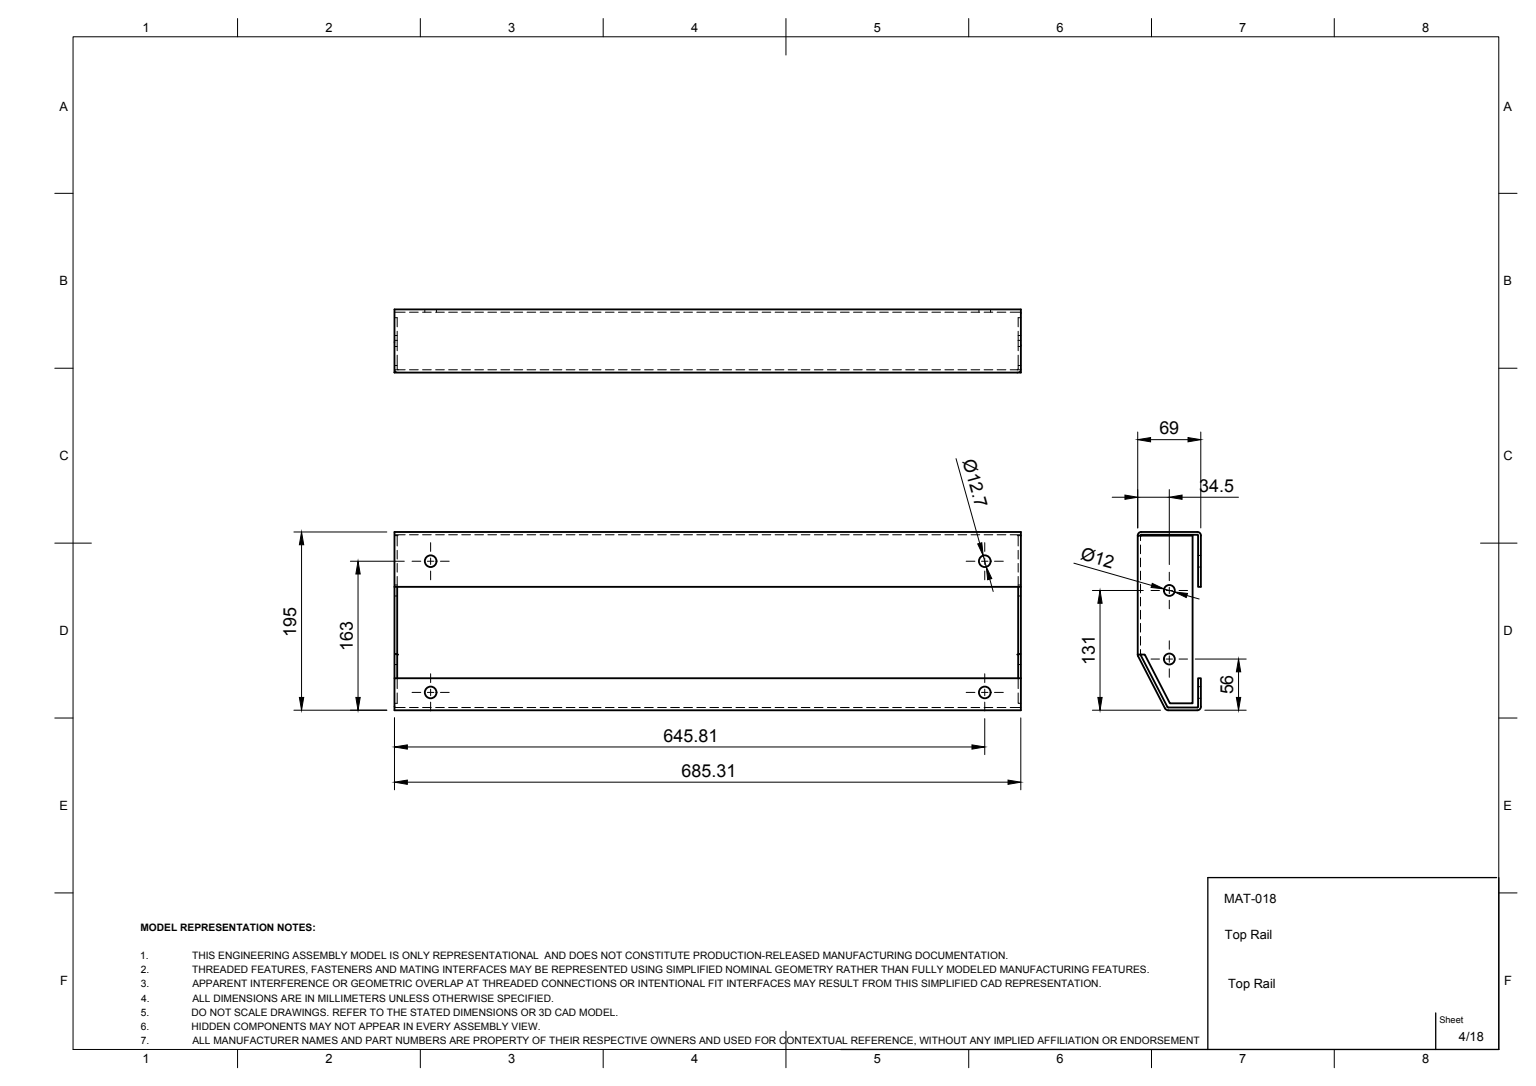
ISO-10303-21;
HEADER;
/* Generated by software containing ST-Developer
 * from STEP Tools, Inc. (www.steptools.com) 
 */

FILE_DESCRIPTION(
/* description */ ('STEP AP214'),
/* implementation_level */ '2;1');

FILE_NAME(
/* name */ 'Top Rail.step',
/* time_stamp */ '2026-11-14T06:16:09-08:00',
/* author */ (''),
/* organization */ (''),
/* preprocessor_version */ 'ST-DEVELOPER v20.2',
/* originating_system */ 'Autodesk Translation Framework v15.17.0.0',
/* authorisation */ '');

FILE_SCHEMA (('AUTOMOTIVE_DESIGN { 1 0 10303 214 3 1 1 }'));
ENDSEC;

DATA;
#10=MECHANICAL_DESIGN_GEOMETRIC_PRESENTATION_REPRESENTATION('',(#348),#18006);
#316=SHAPE_REPRESENTATION_RELATIONSHIP('SRR','None',#18072,#332);
#332=ADVANCED_BREP_SHAPE_REPRESENTATION('',(#364),#17989);
#348=STYLED_ITEM('',(#18170),#364);
#364=MANIFOLD_SOLID_BREP('Body1',#9557);
#401=FACE_BOUND('',#1553,.T.);
#402=FACE_BOUND('',#1554,.T.);
#403=FACE_BOUND('',#1557,.T.);
#404=FACE_BOUND('',#1558,.T.);
#405=FACE_BOUND('',#1568,.T.);
#406=FACE_BOUND('',#1569,.T.);
#407=FACE_BOUND('',#1572,.T.);
#408=FACE_BOUND('',#1573,.T.);
#409=FACE_BOUND('',#1591,.T.);
#410=FACE_BOUND('',#1592,.T.);
#411=FACE_BOUND('',#1594,.T.);
#412=FACE_BOUND('',#1595,.T.);
#413=FACE_BOUND('',#1606,.T.);
#414=FACE_BOUND('',#1607,.T.);
#415=FACE_BOUND('',#1609,.T.);
#416=FACE_BOUND('',#1610,.T.);
#558=PLANE('',#9911);
#559=PLANE('',#9913);
#560=PLANE('',#9915);
#561=PLANE('',#9916);
#562=PLANE('',#9917);
#563=PLANE('',#9919);
#564=PLANE('',#9921);
#565=PLANE('',#9924);
#566=PLANE('',#9925);
#567=PLANE('',#9928);
#568=PLANE('',#9929);
#569=PLANE('',#9932);
#570=PLANE('',#9935);
#571=PLANE('',#9936);
#572=PLANE('',#9939);
#573=PLANE('',#9940);
#574=PLANE('',#9943);
#575=PLANE('',#9946);
#576=PLANE('',#9947);
#577=PLANE('',#9950);
#578=PLANE('',#9951);
#579=PLANE('',#9954);
#580=PLANE('',#9955);
#581=PLANE('',#9958);
#582=PLANE('',#9959);
#583=PLANE('',#9960);
#584=PLANE('',#9961);
#585=PLANE('',#9963);
#586=PLANE('',#9965);
#587=PLANE('',#9968);
#588=PLANE('',#9970);
#589=PLANE('',#9971);
#590=PLANE('',#9972);
#591=PLANE('',#9974);
#592=PLANE('',#9977);
#593=PLANE('',#9979);
#594=PLANE('',#9981);
#595=PLANE('',#9982);
#596=PLANE('',#9983);
#597=PLANE('',#9986);
#598=PLANE('',#9991);
#599=PLANE('',#9992);
#600=PLANE('',#9993);
#601=PLANE('',#9994);
#602=PLANE('',#9995);
#603=PLANE('',#9996);
#604=PLANE('',#9997);
#605=PLANE('',#9998);
#606=PLANE('',#10001);
#607=PLANE('',#10006);
#608=PLANE('',#10007);
#609=PLANE('',#10008);
#610=PLANE('',#10009);
#611=PLANE('',#10010);
#612=PLANE('',#10011);
#613=PLANE('',#10012);
#922=FACE_OUTER_BOUND('',#1520,.T.);
#923=FACE_OUTER_BOUND('',#1521,.T.);
#924=FACE_OUTER_BOUND('',#1522,.T.);
#925=FACE_OUTER_BOUND('',#1523,.T.);
#926=FACE_OUTER_BOUND('',#1524,.T.);
#927=FACE_OUTER_BOUND('',#1525,.T.);
#928=FACE_OUTER_BOUND('',#1526,.T.);
#929=FACE_OUTER_BOUND('',#1527,.T.);
#930=FACE_OUTER_BOUND('',#1528,.T.);
#931=FACE_OUTER_BOUND('',#1529,.T.);
#932=FACE_OUTER_BOUND('',#1530,.T.);
#933=FACE_OUTER_BOUND('',#1531,.T.);
#934=FACE_OUTER_BOUND('',#1532,.T.);
#935=FACE_OUTER_BOUND('',#1533,.T.);
#936=FACE_OUTER_BOUND('',#1534,.T.);
#937=FACE_OUTER_BOUND('',#1535,.T.);
#938=FACE_OUTER_BOUND('',#1536,.T.);
#939=FACE_OUTER_BOUND('',#1537,.T.);
#940=FACE_OUTER_BOUND('',#1538,.T.);
#941=FACE_OUTER_BOUND('',#1539,.T.);
#942=FACE_OUTER_BOUND('',#1540,.T.);
#943=FACE_OUTER_BOUND('',#1541,.T.);
#944=FACE_OUTER_BOUND('',#1542,.T.);
#945=FACE_OUTER_BOUND('',#1543,.T.);
#946=FACE_OUTER_BOUND('',#1544,.T.);
#947=FACE_OUTER_BOUND('',#1545,.T.);
#948=FACE_OUTER_BOUND('',#1546,.T.);
#949=FACE_OUTER_BOUND('',#1547,.T.);
#950=FACE_OUTER_BOUND('',#1548,.T.);
#951=FACE_OUTER_BOUND('',#1549,.T.);
#952=FACE_OUTER_BOUND('',#1550,.T.);
#953=FACE_OUTER_BOUND('',#1551,.T.);
#954=FACE_OUTER_BOUND('',#1552,.T.);
#955=FACE_OUTER_BOUND('',#1555,.T.);
#956=FACE_OUTER_BOUND('',#1556,.T.);
#957=FACE_OUTER_BOUND('',#1559,.T.);
#958=FACE_OUTER_BOUND('',#1560,.T.);
#959=FACE_OUTER_BOUND('',#1561,.T.);
#960=FACE_OUTER_BOUND('',#1562,.T.);
#961=FACE_OUTER_BOUND('',#1563,.T.);
#962=FACE_OUTER_BOUND('',#1564,.T.);
#963=FACE_OUTER_BOUND('',#1565,.T.);
#964=FACE_OUTER_BOUND('',#1566,.T.);
#965=FACE_OUTER_BOUND('',#1567,.T.);
#966=FACE_OUTER_BOUND('',#1570,.T.);
#967=FACE_OUTER_BOUND('',#1571,.T.);
#968=FACE_OUTER_BOUND('',#1574,.T.);
#969=FACE_OUTER_BOUND('',#1575,.T.);
#970=FACE_OUTER_BOUND('',#1576,.T.);
#971=FACE_OUTER_BOUND('',#1577,.T.);
#972=FACE_OUTER_BOUND('',#1578,.T.);
#973=FACE_OUTER_BOUND('',#1579,.T.);
#974=FACE_OUTER_BOUND('',#1580,.T.);
#975=FACE_OUTER_BOUND('',#1581,.T.);
#976=FACE_OUTER_BOUND('',#1582,.T.);
#977=FACE_OUTER_BOUND('',#1583,.T.);
#978=FACE_OUTER_BOUND('',#1584,.T.);
#979=FACE_OUTER_BOUND('',#1585,.T.);
#980=FACE_OUTER_BOUND('',#1586,.T.);
#981=FACE_OUTER_BOUND('',#1587,.T.);
#982=FACE_OUTER_BOUND('',#1588,.T.);
#983=FACE_OUTER_BOUND('',#1589,.T.);
#984=FACE_OUTER_BOUND('',#1590,.T.);
#985=FACE_OUTER_BOUND('',#1593,.T.);
#986=FACE_OUTER_BOUND('',#1596,.T.);
#987=FACE_OUTER_BOUND('',#1597,.T.);
#988=FACE_OUTER_BOUND('',#1598,.T.);
#989=FACE_OUTER_BOUND('',#1599,.T.);
#990=FACE_OUTER_BOUND('',#1600,.T.);
#991=FACE_OUTER_BOUND('',#1601,.T.);
#992=FACE_OUTER_BOUND('',#1602,.T.);
#993=FACE_OUTER_BOUND('',#1603,.T.);
#994=FACE_OUTER_BOUND('',#1604,.T.);
#995=FACE_OUTER_BOUND('',#1605,.T.);
#996=FACE_OUTER_BOUND('',#1608,.T.);
#997=FACE_OUTER_BOUND('',#1611,.T.);
#998=FACE_OUTER_BOUND('',#1612,.T.);
#999=FACE_OUTER_BOUND('',#1613,.T.);
#1520=EDGE_LOOP('',(#6522,#6523,#6524,#6525));
#1521=EDGE_LOOP('',(#6526,#6527,#6528,#6529));
#1522=EDGE_LOOP('',(#6530,#6531,#6532,#6533));
#1523=EDGE_LOOP('',(#6534,#6535,#6536,#6537));
#1524=EDGE_LOOP('',(#6538,#6539,#6540,#6541));
#1525=EDGE_LOOP('',(#6542,#6543,#6544,#6545));
#1526=EDGE_LOOP('',(#6546,#6547,#6548,#6549));
#1527=EDGE_LOOP('',(#6550,#6551,#6552,#6553));
#1528=EDGE_LOOP('',(#6554,#6555,#6556,#6557));
#1529=EDGE_LOOP('',(#6558,#6559,#6560,#6561));
#1530=EDGE_LOOP('',(#6562,#6563,#6564,#6565));
#1531=EDGE_LOOP('',(#6566,#6567,#6568,#6569));
#1532=EDGE_LOOP('',(#6570,#6571,#6572,#6573));
#1533=EDGE_LOOP('',(#6574,#6575,#6576,#6577));
#1534=EDGE_LOOP('',(#6578,#6579,#6580,#6581));
#1535=EDGE_LOOP('',(#6582,#6583,#6584,#6585));
#1536=EDGE_LOOP('',(#6586,#6587,#6588,#6589));
#1537=EDGE_LOOP('',(#6590,#6591,#6592,#6593));
#1538=EDGE_LOOP('',(#6594,#6595,#6596,#6597));
#1539=EDGE_LOOP('',(#6598,#6599,#6600,#6601));
#1540=EDGE_LOOP('',(#6602,#6603,#6604,#6605));
#1541=EDGE_LOOP('',(#6606,#6607,#6608,#6609));
#1542=EDGE_LOOP('',(#6610,#6611,#6612,#6613));
#1543=EDGE_LOOP('',(#6614,#6615,#6616,#6617));
#1544=EDGE_LOOP('',(#6618,#6619,#6620,#6621));
#1545=EDGE_LOOP('',(#6622,#6623,#6624,#6625));
#1546=EDGE_LOOP('',(#6626,#6627,#6628,#6629));
#1547=EDGE_LOOP('',(#6630,#6631,#6632,#6633));
#1548=EDGE_LOOP('',(#6634,#6635,#6636,#6637));
#1549=EDGE_LOOP('',(#6638,#6639,#6640,#6641));
#1550=EDGE_LOOP('',(#6642,#6643,#6644,#6645));
#1551=EDGE_LOOP('',(#6646,#6647,#6648,#6649));
#1552=EDGE_LOOP('',(#6650,#6651,#6652,#6653));
#1553=EDGE_LOOP('',(#6654));
#1554=EDGE_LOOP('',(#6655));
#1555=EDGE_LOOP('',(#6656,#6657,#6658,#6659));
#1556=EDGE_LOOP('',(#6660,#6661,#6662,#6663));
#1557=EDGE_LOOP('',(#6664));
#1558=EDGE_LOOP('',(#6665));
#1559=EDGE_LOOP('',(#6666,#6667,#6668,#6669));
#1560=EDGE_LOOP('',(#6670,#6671,#6672,#6673));
#1561=EDGE_LOOP('',(#6674,#6675,#6676,#6677));
#1562=EDGE_LOOP('',(#6678,#6679,#6680,#6681));
#1563=EDGE_LOOP('',(#6682,#6683,#6684,#6685,#6686,#6687));
#1564=EDGE_LOOP('',(#6688,#6689,#6690,#6691,#6692,#6693));
#1565=EDGE_LOOP('',(#6694,#6695,#6696,#6697));
#1566=EDGE_LOOP('',(#6698,#6699,#6700,#6701));
#1567=EDGE_LOOP('',(#6702,#6703,#6704,#6705));
#1568=EDGE_LOOP('',(#6706));
#1569=EDGE_LOOP('',(#6707));
#1570=EDGE_LOOP('',(#6708,#6709,#6710,#6711));
#1571=EDGE_LOOP('',(#6712,#6713,#6714,#6715));
#1572=EDGE_LOOP('',(#6716));
#1573=EDGE_LOOP('',(#6717));
#1574=EDGE_LOOP('',(#6718,#6719,#6720,#6721));
#1575=EDGE_LOOP('',(#6722,#6723,#6724,#6725));
#1576=EDGE_LOOP('',(#6726,#6727,#6728,#6729,#6730,#6731,#6732,#6733));
#1577=EDGE_LOOP('',(#6734,#6735,#6736,#6737,#6738,#6739,#6740,#6741));
#1578=EDGE_LOOP('',(#6742,#6743,#6744,#6745));
#1579=EDGE_LOOP('',(#6746,#6747,#6748,#6749));
#1580=EDGE_LOOP('',(#6750,#6751,#6752,#6753));
#1581=EDGE_LOOP('',(#6754,#6755,#6756,#6757));
#1582=EDGE_LOOP('',(#6758,#6759,#6760,#6761));
#1583=EDGE_LOOP('',(#6762,#6763,#6764,#6765));
#1584=EDGE_LOOP('',(#6766,#6767,#6768,#6769));
#1585=EDGE_LOOP('',(#6770,#6771,#6772,#6773));
#1586=EDGE_LOOP('',(#6774,#6775,#6776,#6777,#6778,#6779));
#1587=EDGE_LOOP('',(#6780,#6781,#6782,#6783));
#1588=EDGE_LOOP('',(#6784,#6785,#6786,#6787));
#1589=EDGE_LOOP('',(#6788,#6789,#6790,#6791));
#1590=EDGE_LOOP('',(#6792,#6793,#6794,#6795,#6796,#6797));
#1591=EDGE_LOOP('',(#6798));
#1592=EDGE_LOOP('',(#6799));
#1593=EDGE_LOOP('',(#6800,#6801,#6802,#6803,#6804,#6805));
#1594=EDGE_LOOP('',(#6806));
#1595=EDGE_LOOP('',(#6807));
#1596=EDGE_LOOP('',(#6808,#6809,#6810,#6811));
#1597=EDGE_LOOP('',(#6812,#6813,#6814,#6815));
#1598=EDGE_LOOP('',(#6816,#6817,#6818,#6819));
#1599=EDGE_LOOP('',(#6820,#6821,#6822,#6823));
#1600=EDGE_LOOP('',(#6824,#6825,#6826,#6827));
#1601=EDGE_LOOP('',(#6828,#6829,#6830,#6831,#6832,#6833));
#1602=EDGE_LOOP('',(#6834,#6835,#6836,#6837));
#1603=EDGE_LOOP('',(#6838,#6839,#6840,#6841));
#1604=EDGE_LOOP('',(#6842,#6843,#6844,#6845));
#1605=EDGE_LOOP('',(#6846,#6847,#6848,#6849,#6850,#6851));
#1606=EDGE_LOOP('',(#6852));
#1607=EDGE_LOOP('',(#6853));
#1608=EDGE_LOOP('',(#6854,#6855,#6856,#6857,#6858,#6859));
#1609=EDGE_LOOP('',(#6860));
#1610=EDGE_LOOP('',(#6861));
#1611=EDGE_LOOP('',(#6862,#6863,#6864,#6865));
#1612=EDGE_LOOP('',(#6866,#6867,#6868,#6869));
#1613=EDGE_LOOP('',(#6870,#6871,#6872,#6873));
#2247=LINE('',#14188,#2971);
#2248=LINE('',#14194,#2972);
#2249=LINE('',#14200,#2973);
#2250=LINE('',#14206,#2974);
#2251=LINE('',#14212,#2975);
#2252=LINE('',#14218,#2976);
#2253=LINE('',#14224,#2977);
#2254=LINE('',#14230,#2978);
#2255=LINE('',#14235,#2979);
#2256=LINE('',#14239,#2980);
#2257=LINE('',#14240,#2981);
#2258=LINE('',#14244,#2982);
#2259=LINE('',#14248,#2983);
#2260=LINE('',#14249,#2984);
#2261=LINE('',#14252,#2985);
#2262=LINE('',#14253,#2986);
#2263=LINE('',#14255,#2987);
#2264=LINE('',#14256,#2988);
#2265=LINE('',#14260,#2989);
#2266=LINE('',#14262,#2990);
#2267=LINE('',#14264,#2991);
#2268=LINE('',#14265,#2992);
#2269=LINE('',#14269,#2993);
#2270=LINE('',#14272,#2994);
#2271=LINE('',#14273,#2995);
#2272=LINE('',#14276,#2996);
#2273=LINE('',#14280,#2997);
#2274=LINE('',#14281,#2998);
#2275=LINE('',#14285,#2999);
#2276=LINE('',#14289,#3000);
#2277=LINE('',#14293,#3001);
#2278=LINE('',#14295,#3002);
#2279=LINE('',#14296,#3003);
#2280=LINE('',#14300,#3004);
#2281=LINE('',#14304,#3005);
#2282=LINE('',#14308,#3006);
#2283=LINE('',#14310,#3007);
#2284=LINE('',#14311,#3008);
#2285=LINE('',#14318,#3009);
#2286=LINE('',#14322,#3010);
#2287=LINE('',#14323,#3011);
#2288=LINE('',#14327,#3012);
#2289=LINE('',#14332,#3013);
#2290=LINE('',#14334,#3014);
#2291=LINE('',#14335,#3015);
#2292=LINE('',#14340,#3016);
#2293=LINE('',#14345,#3017);
#2294=LINE('',#14350,#3018);
#2295=LINE('',#14352,#3019);
#2296=LINE('',#14353,#3020);
#2297=LINE('',#14357,#3021);
#2298=LINE('',#14361,#3022);
#2299=LINE('',#14364,#3023);
#2300=LINE('',#14365,#3024);
#2301=LINE('',#14369,#3025);
#2302=LINE('',#14374,#3026);
#2303=LINE('',#14376,#3027);
#2304=LINE('',#14377,#3028);
#2305=LINE('',#14381,#3029);
#2306=LINE('',#14385,#3030);
#2307=LINE('',#14388,#3031);
#2308=LINE('',#14389,#3032);
#2309=LINE('',#14392,#3033);
#2310=LINE('',#14393,#3034);
#2311=LINE('',#14394,#3035);
#2312=LINE('',#14397,#3036);
#2313=LINE('',#14398,#3037);
#2314=LINE('',#14400,#3038);
#2315=LINE('',#14401,#3039);
#2316=LINE('',#14403,#3040);
#2317=LINE('',#14405,#3041);
#2318=LINE('',#14407,#3042);
#2319=LINE('',#14409,#3043);
#2320=LINE('',#14412,#3044);
#2321=LINE('',#14414,#3045);
#2322=LINE('',#14416,#3046);
#2323=LINE('',#14419,#3047);
#2324=LINE('',#14420,#3048);
#2325=LINE('',#14423,#3049);
#2326=LINE('',#14424,#3050);
#2327=LINE('',#14426,#3051);
#2328=LINE('',#14427,#3052);
#2329=LINE('',#14429,#3053);
#2330=LINE('',#14431,#3054);
#2331=LINE('',#14433,#3055);
#2332=LINE('',#14434,#3056);
#2333=LINE('',#14436,#3057);
#2334=LINE('',#14437,#3058);
#2335=LINE('',#14438,#3059);
#2336=LINE('',#14440,#3060);
#2337=LINE('',#14442,#3061);
#2338=LINE('',#14444,#3062);
#2339=LINE('',#14452,#3063);
#2340=LINE('',#14459,#3064);
#2341=LINE('',#14461,#3065);
#2342=LINE('',#14463,#3066);
#2343=LINE('',#14466,#3067);
#2344=LINE('',#14468,#3068);
#2345=LINE('',#14469,#3069);
#2346=LINE('',#14472,#3070);
#2347=LINE('',#14474,#3071);
#2348=LINE('',#14475,#3072);
#2349=LINE('',#14478,#3073);
#2350=LINE('',#14480,#3074);
#2351=LINE('',#14481,#3075);
#2352=LINE('',#14484,#3076);
#2353=LINE('',#14486,#3077);
#2354=LINE('',#14487,#3078);
#2355=LINE('',#14489,#3079);
#2356=LINE('',#14491,#3080);
#2357=LINE('',#14498,#3081);
#2358=LINE('',#14504,#3082);
#2359=LINE('',#14506,#3083);
#2360=LINE('',#14508,#3084);
#2361=LINE('',#14511,#3085);
#2362=LINE('',#14513,#3086);
#2363=LINE('',#14514,#3087);
#2364=LINE('',#14517,#3088);
#2365=LINE('',#14519,#3089);
#2366=LINE('',#14520,#3090);
#2367=LINE('',#14523,#3091);
#2368=LINE('',#14525,#3092);
#2369=LINE('',#14526,#3093);
#2370=LINE('',#14529,#3094);
#2371=LINE('',#14531,#3095);
#2372=LINE('',#14532,#3096);
#2373=LINE('',#14534,#3097);
#2374=LINE('',#14536,#3098);
#2971=VECTOR('',#11272,6.00000000000001);
#2972=VECTOR('',#11279,6.00000000000001);
#2973=VECTOR('',#11286,6.00000000000001);
#2974=VECTOR('',#11293,6.00000000000001);
#2975=VECTOR('',#11300,6.34999999999994);
#2976=VECTOR('',#11307,6.34999999999997);
#2977=VECTOR('',#11314,6.34999999999995);
#2978=VECTOR('',#11321,6.34999999999997);
#2979=VECTOR('',#11326,1000.);
#2980=VECTOR('',#11329,1000.);
#2981=VECTOR('',#11330,1000.);
#2982=VECTOR('',#11333,1000.);
#2983=VECTOR('',#11336,1000.);
#2984=VECTOR('',#11337,1000.);
#2985=VECTOR('',#11340,1000.);
#2986=VECTOR('',#11341,1000.);
#2987=VECTOR('',#11342,1000.);
#2988=VECTOR('',#11343,1000.);
#2989=VECTOR('',#11346,1000.);
#2990=VECTOR('',#11347,1000.);
#2991=VECTOR('',#11348,1000.);
#2992=VECTOR('',#11349,1000.);
#2993=VECTOR('',#11352,1000.);
#2994=VECTOR('',#11355,1000.);
#2995=VECTOR('',#11356,1000.);
#2996=VECTOR('',#11359,1000.);
#2997=VECTOR('',#11362,1000.);
#2998=VECTOR('',#11363,1000.);
#2999=VECTOR('',#11366,1000.);
#3000=VECTOR('',#11369,1000.);
#3001=VECTOR('',#11374,1000.);
#3002=VECTOR('',#11375,1000.);
#3003=VECTOR('',#11376,1000.);
#3004=VECTOR('',#11379,1000.);
#3005=VECTOR('',#11382,1000.);
#3006=VECTOR('',#11387,1000.);
#3007=VECTOR('',#11388,1000.);
#3008=VECTOR('',#11389,1000.);
#3009=VECTOR('',#11398,1000.);
#3010=VECTOR('',#11405,1000.);
#3011=VECTOR('',#11406,1000.);
#3012=VECTOR('',#11409,1000.);
#3013=VECTOR('',#11416,1000.);
#3014=VECTOR('',#11417,1000.);
#3015=VECTOR('',#11418,1000.);
#3016=VECTOR('',#11423,1000.);
#3017=VECTOR('',#11428,1000.);
#3018=VECTOR('',#11435,1000.);
#3019=VECTOR('',#11436,1000.);
#3020=VECTOR('',#11437,1000.);
#3021=VECTOR('',#11440,1000.);
#3022=VECTOR('',#11443,1000.);
#3023=VECTOR('',#11448,1000.);
#3024=VECTOR('',#11449,1000.);
#3025=VECTOR('',#11452,1000.);
#3026=VECTOR('',#11459,1000.);
#3027=VECTOR('',#11460,1000.);
#3028=VECTOR('',#11461,1000.);
#3029=VECTOR('',#11464,1000.);
#3030=VECTOR('',#11467,1000.);
#3031=VECTOR('',#11472,1000.);
#3032=VECTOR('',#11473,1000.);
#3033=VECTOR('',#11476,1000.);
#3034=VECTOR('',#11477,1000.);
#3035=VECTOR('',#11478,1000.);
#3036=VECTOR('',#11481,1000.);
#3037=VECTOR('',#11482,1000.);
#3038=VECTOR('',#11485,1000.);
#3039=VECTOR('',#11486,1000.);
#3040=VECTOR('',#11489,1000.);
#3041=VECTOR('',#11492,1000.);
#3042=VECTOR('',#11495,1000.);
#3043=VECTOR('',#11498,1000.);
#3044=VECTOR('',#11503,1000.);
#3045=VECTOR('',#11506,1000.);
#3046=VECTOR('',#11509,1000.);
#3047=VECTOR('',#11512,1000.);
#3048=VECTOR('',#11513,1000.);
#3049=VECTOR('',#11516,1000.);
#3050=VECTOR('',#11517,1000.);
#3051=VECTOR('',#11520,1000.);
#3052=VECTOR('',#11521,1000.);
#3053=VECTOR('',#11524,1000.);
#3054=VECTOR('',#11527,1000.);
#3055=VECTOR('',#11530,1000.);
#3056=VECTOR('',#11531,1000.);
#3057=VECTOR('',#11534,1000.);
#3058=VECTOR('',#11535,1000.);
#3059=VECTOR('',#11536,1000.);
#3060=VECTOR('',#11539,1000.);
#3061=VECTOR('',#11542,1000.);
#3062=VECTOR('',#11545,1000.);
#3063=VECTOR('',#11556,1000.);
#3064=VECTOR('',#11565,1000.);
#3065=VECTOR('',#11568,1000.);
#3066=VECTOR('',#11571,1000.);
#3067=VECTOR('',#11574,1000.);
#3068=VECTOR('',#11575,1000.);
#3069=VECTOR('',#11576,1000.);
#3070=VECTOR('',#11579,1000.);
#3071=VECTOR('',#11580,1000.);
#3072=VECTOR('',#11581,1000.);
#3073=VECTOR('',#11584,1000.);
#3074=VECTOR('',#11585,1000.);
#3075=VECTOR('',#11586,1000.);
#3076=VECTOR('',#11589,1000.);
#3077=VECTOR('',#11590,1000.);
#3078=VECTOR('',#11591,1000.);
#3079=VECTOR('',#11594,1000.);
#3080=VECTOR('',#11597,1000.);
#3081=VECTOR('',#11606,1000.);
#3082=VECTOR('',#11613,1000.);
#3083=VECTOR('',#11616,1000.);
#3084=VECTOR('',#11619,1000.);
#3085=VECTOR('',#11622,1000.);
#3086=VECTOR('',#11623,1000.);
#3087=VECTOR('',#11624,1000.);
#3088=VECTOR('',#11627,1000.);
#3089=VECTOR('',#11628,1000.);
#3090=VECTOR('',#11629,1000.);
#3091=VECTOR('',#11632,1000.);
#3092=VECTOR('',#11633,1000.);
#3093=VECTOR('',#11634,1000.);
#3094=VECTOR('',#11637,1000.);
#3095=VECTOR('',#11638,1000.);
#3096=VECTOR('',#11639,1000.);
#3097=VECTOR('',#11642,1000.);
#3098=VECTOR('',#11645,1000.);
#3618=CIRCLE('',#9888,6.00000000000001);
#3619=CIRCLE('',#9889,6.00000000000001);
#3620=CIRCLE('',#9891,6.00000000000002);
#3621=CIRCLE('',#9892,6.00000000000001);
#3622=CIRCLE('',#9894,6.00000000000001);
#3623=CIRCLE('',#9895,6.00000000000001);
#3624=CIRCLE('',#9897,6.00000000000001);
#3625=CIRCLE('',#9898,6.00000000000002);
#3626=CIRCLE('',#9900,6.34999999999994);
#3627=CIRCLE('',#9901,6.34999999999994);
#3628=CIRCLE('',#9903,6.34999999999994);
#3629=CIRCLE('',#9904,6.34999999999997);
#3630=CIRCLE('',#9906,6.34999999999995);
#3631=CIRCLE('',#9907,6.34999999999995);
#3632=CIRCLE('',#9909,6.34999999999997);
#3633=CIRCLE('',#9910,6.34999999999997);
#3634=CIRCLE('',#9912,4.);
#3635=CIRCLE('',#9914,4.);
#3636=CIRCLE('',#9918,4.);
#3637=CIRCLE('',#9920,4.);
#3638=CIRCLE('',#9922,4.);
#3639=CIRCLE('',#9923,1.);
#3640=CIRCLE('',#9926,4.);
#3641=CIRCLE('',#9927,1.);
#3642=CIRCLE('',#9930,4.);
#3643=CIRCLE('',#9931,1.);
#3644=CIRCLE('',#9933,4.);
#3645=CIRCLE('',#9934,1.);
#3646=CIRCLE('',#9937,4.);
#3647=CIRCLE('',#9938,1.);
#3648=CIRCLE('',#9941,4.);
#3649=CIRCLE('',#9942,1.);
#3650=CIRCLE('',#9944,4.);
#3651=CIRCLE('',#9945,1.);
#3652=CIRCLE('',#9948,4.);
#3653=CIRCLE('',#9949,1.);
#3654=CIRCLE('',#9952,4.);
#3655=CIRCLE('',#9953,1.);
#3656=CIRCLE('',#9956,4.);
#3657=CIRCLE('',#9957,1.);
#3658=CIRCLE('',#9984,4.);
#3659=CIRCLE('',#9985,1.);
#3660=CIRCLE('',#9987,4.);
#3661=CIRCLE('',#9988,1.);
#3662=CIRCLE('',#9999,1.);
#3663=CIRCLE('',#10000,4.);
#3664=CIRCLE('',#10002,4.);
#3665=CIRCLE('',#10003,1.);
#4119=VERTEX_POINT('',#14185);
#4120=VERTEX_POINT('',#14187);
#4121=VERTEX_POINT('',#14191);
#4122=VERTEX_POINT('',#14193);
#4123=VERTEX_POINT('',#14197);
#4124=VERTEX_POINT('',#14199);
#4125=VERTEX_POINT('',#14203);
#4126=VERTEX_POINT('',#14205);
#4127=VERTEX_POINT('',#14209);
#4128=VERTEX_POINT('',#14211);
#4129=VERTEX_POINT('',#14215);
#4130=VERTEX_POINT('',#14217);
#4131=VERTEX_POINT('',#14221);
#4132=VERTEX_POINT('',#14223);
#4133=VERTEX_POINT('',#14227);
#4134=VERTEX_POINT('',#14229);
#4135=VERTEX_POINT('',#14233);
#4136=VERTEX_POINT('',#14234);
#4137=VERTEX_POINT('',#14236);
#4138=VERTEX_POINT('',#14238);
#4139=VERTEX_POINT('',#14242);
#4140=VERTEX_POINT('',#14243);
#4141=VERTEX_POINT('',#14245);
#4142=VERTEX_POINT('',#14247);
#4143=VERTEX_POINT('',#14251);
#4144=VERTEX_POINT('',#14254);
#4145=VERTEX_POINT('',#14258);
#4146=VERTEX_POINT('',#14259);
#4147=VERTEX_POINT('',#14261);
#4148=VERTEX_POINT('',#14263);
#4149=VERTEX_POINT('',#14267);
#4150=VERTEX_POINT('',#14268);
#4151=VERTEX_POINT('',#14271);
#4152=VERTEX_POINT('',#14275);
#4153=VERTEX_POINT('',#14277);
#4154=VERTEX_POINT('',#14279);
#4155=VERTEX_POINT('',#14283);
#4156=VERTEX_POINT('',#14284);
#4157=VERTEX_POINT('',#14286);
#4158=VERTEX_POINT('',#14288);
#4159=VERTEX_POINT('',#14292);
#4160=VERTEX_POINT('',#14294);
#4161=VERTEX_POINT('',#14298);
#4162=VERTEX_POINT('',#14299);
#4163=VERTEX_POINT('',#14301);
#4164=VERTEX_POINT('',#14303);
#4165=VERTEX_POINT('',#14307);
#4166=VERTEX_POINT('',#14309);
#4167=VERTEX_POINT('',#14316);
#4168=VERTEX_POINT('',#14317);
#4169=VERTEX_POINT('',#14325);
#4170=VERTEX_POINT('',#14326);
#4171=VERTEX_POINT('',#14331);
#4172=VERTEX_POINT('',#14333);
#4173=VERTEX_POINT('',#14337);
#4174=VERTEX_POINT('',#14339);
#4175=VERTEX_POINT('',#14343);
#4176=VERTEX_POINT('',#14344);
#4177=VERTEX_POINT('',#14349);
#4178=VERTEX_POINT('',#14351);
#4179=VERTEX_POINT('',#14355);
#4180=VERTEX_POINT('',#14356);
#4181=VERTEX_POINT('',#14358);
#4182=VERTEX_POINT('',#14360);
#4183=VERTEX_POINT('',#14367);
#4184=VERTEX_POINT('',#14368);
#4185=VERTEX_POINT('',#14373);
#4186=VERTEX_POINT('',#14375);
#4187=VERTEX_POINT('',#14379);
#4188=VERTEX_POINT('',#14380);
#4189=VERTEX_POINT('',#14382);
#4190=VERTEX_POINT('',#14384);
#4191=VERTEX_POINT('',#14391);
#4192=VERTEX_POINT('',#14396);
#4193=VERTEX_POINT('',#14418);
#4194=VERTEX_POINT('',#14422);
#4195=VERTEX_POINT('',#14449);
#4196=VERTEX_POINT('',#14451);
#4197=VERTEX_POINT('',#14455);
#4198=VERTEX_POINT('',#14457);
#4199=VERTEX_POINT('',#14465);
#4200=VERTEX_POINT('',#14467);
#4201=VERTEX_POINT('',#14471);
#4202=VERTEX_POINT('',#14473);
#4203=VERTEX_POINT('',#14477);
#4204=VERTEX_POINT('',#14479);
#4205=VERTEX_POINT('',#14483);
#4206=VERTEX_POINT('',#14485);
#4207=VERTEX_POINT('',#14494);
#4208=VERTEX_POINT('',#14496);
#4209=VERTEX_POINT('',#14500);
#4210=VERTEX_POINT('',#14502);
#4211=VERTEX_POINT('',#14510);
#4212=VERTEX_POINT('',#14512);
#4213=VERTEX_POINT('',#14516);
#4214=VERTEX_POINT('',#14518);
#4215=VERTEX_POINT('',#14522);
#4216=VERTEX_POINT('',#14524);
#4217=VERTEX_POINT('',#14528);
#4218=VERTEX_POINT('',#14530);
#5009=EDGE_CURVE('',#4119,#4119,#3618,.T.);
#5010=EDGE_CURVE('',#4119,#4120,#2247,.T.);
#5011=EDGE_CURVE('',#4120,#4120,#3619,.T.);
#5012=EDGE_CURVE('',#4121,#4121,#3620,.T.);
#5013=EDGE_CURVE('',#4121,#4122,#2248,.T.);
#5014=EDGE_CURVE('',#4122,#4122,#3621,.T.);
#5015=EDGE_CURVE('',#4123,#4123,#3622,.T.);
#5016=EDGE_CURVE('',#4123,#4124,#2249,.T.);
#5017=EDGE_CURVE('',#4124,#4124,#3623,.T.);
#5018=EDGE_CURVE('',#4125,#4125,#3624,.T.);
#5019=EDGE_CURVE('',#4125,#4126,#2250,.T.);
#5020=EDGE_CURVE('',#4126,#4126,#3625,.T.);
#5021=EDGE_CURVE('',#4127,#4127,#3626,.T.);
#5022=EDGE_CURVE('',#4127,#4128,#2251,.T.);
#5023=EDGE_CURVE('',#4128,#4128,#3627,.T.);
#5024=EDGE_CURVE('',#4129,#4129,#3628,.T.);
#5025=EDGE_CURVE('',#4129,#4130,#2252,.T.);
#5026=EDGE_CURVE('',#4130,#4130,#3629,.T.);
#5027=EDGE_CURVE('',#4131,#4131,#3630,.T.);
#5028=EDGE_CURVE('',#4131,#4132,#2253,.T.);
#5029=EDGE_CURVE('',#4132,#4132,#3631,.T.);
#5030=EDGE_CURVE('',#4133,#4133,#3632,.T.);
#5031=EDGE_CURVE('',#4133,#4134,#2254,.T.);
#5032=EDGE_CURVE('',#4134,#4134,#3633,.T.);
#5033=EDGE_CURVE('',#4135,#4136,#2255,.T.);
#5034=EDGE_CURVE('',#4136,#4137,#3634,.T.);
#5035=EDGE_CURVE('',#4138,#4137,#2256,.T.);
#5036=EDGE_CURVE('',#4138,#4135,#2257,.T.);
#5037=EDGE_CURVE('',#4139,#4140,#2258,.T.);
#5038=EDGE_CURVE('',#4139,#4141,#3635,.T.);
#5039=EDGE_CURVE('',#4141,#4142,#2259,.T.);
#5040=EDGE_CURVE('',#4142,#4140,#2260,.T.);
#5041=EDGE_CURVE('',#4143,#4137,#2261,.T.);
#5042=EDGE_CURVE('',#4137,#4139,#2262,.T.);
#5043=EDGE_CURVE('',#4144,#4139,#2263,.T.);
#5044=EDGE_CURVE('',#4144,#4143,#2264,.T.);
#5045=EDGE_CURVE('',#4145,#4146,#2265,.T.);
#5046=EDGE_CURVE('',#4147,#4145,#2266,.T.);
#5047=EDGE_CURVE('',#4148,#4147,#2267,.T.);
#5048=EDGE_CURVE('',#4148,#4146,#2268,.T.);
#5049=EDGE_CURVE('',#4149,#4150,#2269,.T.);
#5050=EDGE_CURVE('',#4150,#4144,#3636,.T.);
#5051=EDGE_CURVE('',#4151,#4144,#2270,.T.);
#5052=EDGE_CURVE('',#4151,#4149,#2271,.T.);
#5053=EDGE_CURVE('',#4152,#4143,#2272,.T.);
#5054=EDGE_CURVE('',#4143,#4153,#3637,.T.);
#5055=EDGE_CURVE('',#4154,#4153,#2273,.T.);
#5056=EDGE_CURVE('',#4154,#4152,#2274,.T.);
#5057=EDGE_CURVE('',#4155,#4156,#2275,.T.);
#5058=EDGE_CURVE('',#4157,#4155,#3638,.T.);
#5059=EDGE_CURVE('',#4158,#4157,#2276,.T.);
#5060=EDGE_CURVE('',#4158,#4156,#3639,.T.);
#5061=EDGE_CURVE('',#4155,#4159,#2277,.T.);
#5062=EDGE_CURVE('',#4156,#4160,#2278,.T.);
#5063=EDGE_CURVE('',#4160,#4159,#2279,.T.);
#5064=EDGE_CURVE('',#4161,#4162,#2280,.T.);
#5065=EDGE_CURVE('',#4161,#4163,#3640,.T.);
#5066=EDGE_CURVE('',#4164,#4163,#2281,.T.);
#5067=EDGE_CURVE('',#4162,#4164,#3641,.T.);
#5068=EDGE_CURVE('',#4165,#4161,#2282,.T.);
#5069=EDGE_CURVE('',#4166,#4162,#2283,.T.);
#5070=EDGE_CURVE('',#4166,#4165,#2284,.T.);
#5071=EDGE_CURVE('',#4159,#4151,#3642,.T.);
#5072=EDGE_CURVE('',#4160,#4149,#3643,.T.);
#5073=EDGE_CURVE('',#4167,#4168,#2285,.T.);
#5074=EDGE_CURVE('',#4167,#4140,#3644,.T.);
#5075=EDGE_CURVE('',#4168,#4142,#3645,.T.);
#5076=EDGE_CURVE('',#4163,#4167,#2286,.T.);
#5077=EDGE_CURVE('',#4164,#4168,#2287,.T.);
#5078=EDGE_CURVE('',#4169,#4170,#2288,.T.);
#5079=EDGE_CURVE('',#4152,#4169,#3646,.T.);
#5080=EDGE_CURVE('',#4154,#4170,#3647,.T.);
#5081=EDGE_CURVE('',#4169,#4171,#2289,.T.);
#5082=EDGE_CURVE('',#4170,#4172,#2290,.T.);
#5083=EDGE_CURVE('',#4172,#4171,#2291,.T.);
#5084=EDGE_CURVE('',#4138,#4173,#3648,.T.);
#5085=EDGE_CURVE('',#4174,#4173,#2292,.T.);
#5086=EDGE_CURVE('',#4135,#4174,#3649,.T.);
#5087=EDGE_CURVE('',#4175,#4176,#2293,.T.);
#5088=EDGE_CURVE('',#4171,#4175,#3650,.T.);
#5089=EDGE_CURVE('',#4172,#4176,#3651,.T.);
#5090=EDGE_CURVE('',#4175,#4177,#2294,.T.);
#5091=EDGE_CURVE('',#4176,#4178,#2295,.T.);
#5092=EDGE_CURVE('',#4178,#4177,#2296,.T.);
#5093=EDGE_CURVE('',#4179,#4180,#2297,.T.);
#5094=EDGE_CURVE('',#4179,#4181,#3652,.T.);
#5095=EDGE_CURVE('',#4182,#4181,#2298,.T.);
#5096=EDGE_CURVE('',#4180,#4182,#3653,.T.);
#5097=EDGE_CURVE('',#4173,#4179,#2299,.T.);
#5098=EDGE_CURVE('',#4174,#4180,#2300,.T.);
#5099=EDGE_CURVE('',#4183,#4184,#2301,.T.);
#5100=EDGE_CURVE('',#4177,#4183,#3654,.T.);
#5101=EDGE_CURVE('',#4178,#4184,#3655,.T.);
#5102=EDGE_CURVE('',#4183,#4185,#2302,.T.);
#5103=EDGE_CURVE('',#4184,#4186,#2303,.T.);
#5104=EDGE_CURVE('',#4185,#4186,#2304,.T.);
#5105=EDGE_CURVE('',#4187,#4188,#2305,.T.);
#5106=EDGE_CURVE('',#4187,#4189,#3656,.T.);
#5107=EDGE_CURVE('',#4190,#4189,#2306,.T.);
#5108=EDGE_CURVE('',#4188,#4190,#3657,.T.);
#5109=EDGE_CURVE('',#4181,#4187,#2307,.T.);
#5110=EDGE_CURVE('',#4182,#4188,#2308,.T.);
#5111=EDGE_CURVE('',#4190,#4191,#2309,.T.);
#5112=EDGE_CURVE('',#4186,#4191,#2310,.T.);
#5113=EDGE_CURVE('',#4184,#4190,#2311,.T.);
#5114=EDGE_CURVE('',#4192,#4191,#2312,.T.);
#5115=EDGE_CURVE('',#4185,#4192,#2313,.T.);
#5116=EDGE_CURVE('',#4189,#4192,#2314,.T.);
#5117=EDGE_CURVE('',#4183,#4189,#2315,.T.);
#5118=EDGE_CURVE('',#4177,#4187,#2316,.T.);
#5119=EDGE_CURVE('',#4175,#4181,#2317,.T.);
#5120=EDGE_CURVE('',#4171,#4179,#2318,.T.);
#5121=EDGE_CURVE('',#4169,#4173,#2319,.T.);
#5122=EDGE_CURVE('',#4159,#4167,#2320,.T.);
#5123=EDGE_CURVE('',#4155,#4163,#2321,.T.);
#5124=EDGE_CURVE('',#4157,#4161,#2322,.T.);
#5125=EDGE_CURVE('',#4193,#4165,#2323,.T.);
#5126=EDGE_CURVE('',#4193,#4157,#2324,.T.);
#5127=EDGE_CURVE('',#4194,#4166,#2325,.T.);
#5128=EDGE_CURVE('',#4194,#4193,#2326,.T.);
#5129=EDGE_CURVE('',#4158,#4162,#2327,.T.);
#5130=EDGE_CURVE('',#4194,#4158,#2328,.T.);
#5131=EDGE_CURVE('',#4156,#4164,#2329,.T.);
#5132=EDGE_CURVE('',#4160,#4168,#2330,.T.);
#5133=EDGE_CURVE('',#4146,#4141,#2331,.T.);
#5134=EDGE_CURVE('',#4150,#4148,#2332,.T.);
#5135=EDGE_CURVE('',#4170,#4174,#2333,.T.);
#5136=EDGE_CURVE('',#4153,#4147,#2334,.T.);
#5137=EDGE_CURVE('',#4136,#4145,#2335,.T.);
#5138=EDGE_CURVE('',#4172,#4180,#2336,.T.);
#5139=EDGE_CURVE('',#4176,#4182,#2337,.T.);
#5140=EDGE_CURVE('',#4178,#4188,#2338,.T.);
#5141=EDGE_CURVE('',#4153,#4195,#3658,.T.);
#5142=EDGE_CURVE('',#4196,#4195,#2339,.T.);
#5143=EDGE_CURVE('',#4147,#4196,#3659,.T.);
#5144=EDGE_CURVE('',#4197,#4150,#3660,.T.);
#5145=EDGE_CURVE('',#4198,#4148,#3661,.T.);
#5146=EDGE_CURVE('',#4198,#4197,#2340,.T.);
#5147=EDGE_CURVE('',#4197,#4195,#2341,.T.);
#5148=EDGE_CURVE('',#4196,#4198,#2342,.T.);
#5149=EDGE_CURVE('',#4198,#4199,#2343,.T.);
#5150=EDGE_CURVE('',#4200,#4199,#2344,.T.);
#5151=EDGE_CURVE('',#4197,#4200,#2345,.T.);
#5152=EDGE_CURVE('',#4201,#4195,#2346,.T.);
#5153=EDGE_CURVE('',#4202,#4201,#2347,.T.);
#5154=EDGE_CURVE('',#4202,#4196,#2348,.T.);
#5155=EDGE_CURVE('',#4200,#4203,#2349,.T.);
#5156=EDGE_CURVE('',#4203,#4204,#2350,.T.);
#5157=EDGE_CURVE('',#4204,#4201,#2351,.T.);
#5158=EDGE_CURVE('',#4205,#4202,#2352,.T.);
#5159=EDGE_CURVE('',#4206,#4205,#2353,.T.);
#5160=EDGE_CURVE('',#4199,#4206,#2354,.T.);
#5161=EDGE_CURVE('',#4206,#4203,#2355,.T.);
#5162=EDGE_CURVE('',#4205,#4204,#2356,.T.);
#5163=EDGE_CURVE('',#4146,#4207,#3662,.T.);
#5164=EDGE_CURVE('',#4141,#4208,#3663,.T.);
#5165=EDGE_CURVE('',#4207,#4208,#2357,.T.);
#5166=EDGE_CURVE('',#4209,#4136,#3664,.T.);
#5167=EDGE_CURVE('',#4210,#4145,#3665,.T.);
#5168=EDGE_CURVE('',#4210,#4209,#2358,.T.);
#5169=EDGE_CURVE('',#4209,#4208,#2359,.T.);
#5170=EDGE_CURVE('',#4207,#4210,#2360,.T.);
#5171=EDGE_CURVE('',#4211,#4208,#2361,.T.);
#5172=EDGE_CURVE('',#4211,#4212,#2362,.T.);
#5173=EDGE_CURVE('',#4212,#4207,#2363,.T.);
#5174=EDGE_CURVE('',#4210,#4213,#2364,.T.);
#5175=EDGE_CURVE('',#4213,#4214,#2365,.T.);
#5176=EDGE_CURVE('',#4209,#4214,#2366,.T.);
#5177=EDGE_CURVE('',#4214,#4215,#2367,.T.);
#5178=EDGE_CURVE('',#4215,#4216,#2368,.T.);
#5179=EDGE_CURVE('',#4216,#4211,#2369,.T.);
#5180=EDGE_CURVE('',#4217,#4212,#2370,.T.);
#5181=EDGE_CURVE('',#4218,#4217,#2371,.T.);
#5182=EDGE_CURVE('',#4213,#4218,#2372,.T.);
#5183=EDGE_CURVE('',#4217,#4216,#2373,.T.);
#5184=EDGE_CURVE('',#4218,#4215,#2374,.T.);
#6522=ORIENTED_EDGE('',*,*,#5009,.T.);
#6523=ORIENTED_EDGE('',*,*,#5010,.T.);
#6524=ORIENTED_EDGE('',*,*,#5011,.T.);
#6525=ORIENTED_EDGE('',*,*,#5010,.F.);
#6526=ORIENTED_EDGE('',*,*,#5012,.T.);
#6527=ORIENTED_EDGE('',*,*,#5013,.T.);
#6528=ORIENTED_EDGE('',*,*,#5014,.T.);
#6529=ORIENTED_EDGE('',*,*,#5013,.F.);
#6530=ORIENTED_EDGE('',*,*,#5015,.F.);
#6531=ORIENTED_EDGE('',*,*,#5016,.T.);
#6532=ORIENTED_EDGE('',*,*,#5017,.T.);
#6533=ORIENTED_EDGE('',*,*,#5016,.F.);
#6534=ORIENTED_EDGE('',*,*,#5018,.F.);
#6535=ORIENTED_EDGE('',*,*,#5019,.T.);
#6536=ORIENTED_EDGE('',*,*,#5020,.T.);
#6537=ORIENTED_EDGE('',*,*,#5019,.F.);
#6538=ORIENTED_EDGE('',*,*,#5021,.F.);
#6539=ORIENTED_EDGE('',*,*,#5022,.T.);
#6540=ORIENTED_EDGE('',*,*,#5023,.T.);
#6541=ORIENTED_EDGE('',*,*,#5022,.F.);
#6542=ORIENTED_EDGE('',*,*,#5024,.F.);
#6543=ORIENTED_EDGE('',*,*,#5025,.T.);
#6544=ORIENTED_EDGE('',*,*,#5026,.T.);
#6545=ORIENTED_EDGE('',*,*,#5025,.F.);
#6546=ORIENTED_EDGE('',*,*,#5027,.F.);
#6547=ORIENTED_EDGE('',*,*,#5028,.T.);
#6548=ORIENTED_EDGE('',*,*,#5029,.T.);
#6549=ORIENTED_EDGE('',*,*,#5028,.F.);
#6550=ORIENTED_EDGE('',*,*,#5030,.F.);
#6551=ORIENTED_EDGE('',*,*,#5031,.T.);
#6552=ORIENTED_EDGE('',*,*,#5032,.T.);
#6553=ORIENTED_EDGE('',*,*,#5031,.F.);
#6554=ORIENTED_EDGE('',*,*,#5033,.T.);
#6555=ORIENTED_EDGE('',*,*,#5034,.T.);
#6556=ORIENTED_EDGE('',*,*,#5035,.F.);
#6557=ORIENTED_EDGE('',*,*,#5036,.T.);
#6558=ORIENTED_EDGE('',*,*,#5037,.F.);
#6559=ORIENTED_EDGE('',*,*,#5038,.T.);
#6560=ORIENTED_EDGE('',*,*,#5039,.T.);
#6561=ORIENTED_EDGE('',*,*,#5040,.T.);
#6562=ORIENTED_EDGE('',*,*,#5041,.T.);
#6563=ORIENTED_EDGE('',*,*,#5042,.T.);
#6564=ORIENTED_EDGE('',*,*,#5043,.F.);
#6565=ORIENTED_EDGE('',*,*,#5044,.T.);
#6566=ORIENTED_EDGE('',*,*,#5045,.F.);
#6567=ORIENTED_EDGE('',*,*,#5046,.F.);
#6568=ORIENTED_EDGE('',*,*,#5047,.F.);
#6569=ORIENTED_EDGE('',*,*,#5048,.T.);
#6570=ORIENTED_EDGE('',*,*,#5049,.T.);
#6571=ORIENTED_EDGE('',*,*,#5050,.T.);
#6572=ORIENTED_EDGE('',*,*,#5051,.F.);
#6573=ORIENTED_EDGE('',*,*,#5052,.T.);
#6574=ORIENTED_EDGE('',*,*,#5053,.T.);
#6575=ORIENTED_EDGE('',*,*,#5054,.T.);
#6576=ORIENTED_EDGE('',*,*,#5055,.F.);
#6577=ORIENTED_EDGE('',*,*,#5056,.T.);
#6578=ORIENTED_EDGE('',*,*,#5057,.F.);
#6579=ORIENTED_EDGE('',*,*,#5058,.F.);
#6580=ORIENTED_EDGE('',*,*,#5059,.F.);
#6581=ORIENTED_EDGE('',*,*,#5060,.T.);
#6582=ORIENTED_EDGE('',*,*,#5061,.F.);
#6583=ORIENTED_EDGE('',*,*,#5057,.T.);
#6584=ORIENTED_EDGE('',*,*,#5062,.T.);
#6585=ORIENTED_EDGE('',*,*,#5063,.T.);
#6586=ORIENTED_EDGE('',*,*,#5064,.F.);
#6587=ORIENTED_EDGE('',*,*,#5065,.T.);
#6588=ORIENTED_EDGE('',*,*,#5066,.F.);
#6589=ORIENTED_EDGE('',*,*,#5067,.F.);
#6590=ORIENTED_EDGE('',*,*,#5068,.T.);
#6591=ORIENTED_EDGE('',*,*,#5064,.T.);
#6592=ORIENTED_EDGE('',*,*,#5069,.F.);
#6593=ORIENTED_EDGE('',*,*,#5070,.T.);
#6594=ORIENTED_EDGE('',*,*,#5052,.F.);
#6595=ORIENTED_EDGE('',*,*,#5071,.F.);
#6596=ORIENTED_EDGE('',*,*,#5063,.F.);
#6597=ORIENTED_EDGE('',*,*,#5072,.T.);
#6598=ORIENTED_EDGE('',*,*,#5073,.F.);
#6599=ORIENTED_EDGE('',*,*,#5074,.T.);
#6600=ORIENTED_EDGE('',*,*,#5040,.F.);
#6601=ORIENTED_EDGE('',*,*,#5075,.F.);
#6602=ORIENTED_EDGE('',*,*,#5076,.T.);
#6603=ORIENTED_EDGE('',*,*,#5073,.T.);
#6604=ORIENTED_EDGE('',*,*,#5077,.F.);
#6605=ORIENTED_EDGE('',*,*,#5066,.T.);
#6606=ORIENTED_EDGE('',*,*,#5078,.F.);
#6607=ORIENTED_EDGE('',*,*,#5079,.F.);
#6608=ORIENTED_EDGE('',*,*,#5056,.F.);
#6609=ORIENTED_EDGE('',*,*,#5080,.T.);
#6610=ORIENTED_EDGE('',*,*,#5081,.F.);
#6611=ORIENTED_EDGE('',*,*,#5078,.T.);
#6612=ORIENTED_EDGE('',*,*,#5082,.T.);
#6613=ORIENTED_EDGE('',*,*,#5083,.T.);
#6614=ORIENTED_EDGE('',*,*,#5036,.F.);
#6615=ORIENTED_EDGE('',*,*,#5084,.T.);
#6616=ORIENTED_EDGE('',*,*,#5085,.F.);
#6617=ORIENTED_EDGE('',*,*,#5086,.F.);
#6618=ORIENTED_EDGE('',*,*,#5087,.F.);
#6619=ORIENTED_EDGE('',*,*,#5088,.F.);
#6620=ORIENTED_EDGE('',*,*,#5083,.F.);
#6621=ORIENTED_EDGE('',*,*,#5089,.T.);
#6622=ORIENTED_EDGE('',*,*,#5090,.F.);
#6623=ORIENTED_EDGE('',*,*,#5087,.T.);
#6624=ORIENTED_EDGE('',*,*,#5091,.T.);
#6625=ORIENTED_EDGE('',*,*,#5092,.T.);
#6626=ORIENTED_EDGE('',*,*,#5093,.F.);
#6627=ORIENTED_EDGE('',*,*,#5094,.T.);
#6628=ORIENTED_EDGE('',*,*,#5095,.F.);
#6629=ORIENTED_EDGE('',*,*,#5096,.F.);
#6630=ORIENTED_EDGE('',*,*,#5097,.T.);
#6631=ORIENTED_EDGE('',*,*,#5093,.T.);
#6632=ORIENTED_EDGE('',*,*,#5098,.F.);
#6633=ORIENTED_EDGE('',*,*,#5085,.T.);
#6634=ORIENTED_EDGE('',*,*,#5099,.F.);
#6635=ORIENTED_EDGE('',*,*,#5100,.F.);
#6636=ORIENTED_EDGE('',*,*,#5092,.F.);
#6637=ORIENTED_EDGE('',*,*,#5101,.T.);
#6638=ORIENTED_EDGE('',*,*,#5102,.F.);
#6639=ORIENTED_EDGE('',*,*,#5099,.T.);
#6640=ORIENTED_EDGE('',*,*,#5103,.T.);
#6641=ORIENTED_EDGE('',*,*,#5104,.F.);
#6642=ORIENTED_EDGE('',*,*,#5105,.F.);
#6643=ORIENTED_EDGE('',*,*,#5106,.T.);
#6644=ORIENTED_EDGE('',*,*,#5107,.F.);
#6645=ORIENTED_EDGE('',*,*,#5108,.F.);
#6646=ORIENTED_EDGE('',*,*,#5109,.T.);
#6647=ORIENTED_EDGE('',*,*,#5105,.T.);
#6648=ORIENTED_EDGE('',*,*,#5110,.F.);
#6649=ORIENTED_EDGE('',*,*,#5095,.T.);
#6650=ORIENTED_EDGE('',*,*,#5111,.T.);
#6651=ORIENTED_EDGE('',*,*,#5112,.F.);
#6652=ORIENTED_EDGE('',*,*,#5103,.F.);
#6653=ORIENTED_EDGE('',*,*,#5113,.T.);
#6654=ORIENTED_EDGE('',*,*,#5021,.T.);
#6655=ORIENTED_EDGE('',*,*,#5024,.T.);
#6656=ORIENTED_EDGE('',*,*,#5114,.F.);
#6657=ORIENTED_EDGE('',*,*,#5115,.F.);
#6658=ORIENTED_EDGE('',*,*,#5104,.T.);
#6659=ORIENTED_EDGE('',*,*,#5112,.T.);
#6660=ORIENTED_EDGE('',*,*,#5116,.F.);
#6661=ORIENTED_EDGE('',*,*,#5117,.F.);
#6662=ORIENTED_EDGE('',*,*,#5102,.T.);
#6663=ORIENTED_EDGE('',*,*,#5115,.T.);
#6664=ORIENTED_EDGE('',*,*,#5023,.F.);
#6665=ORIENTED_EDGE('',*,*,#5026,.F.);
#6666=ORIENTED_EDGE('',*,*,#5106,.F.);
#6667=ORIENTED_EDGE('',*,*,#5118,.F.);
#6668=ORIENTED_EDGE('',*,*,#5100,.T.);
#6669=ORIENTED_EDGE('',*,*,#5117,.T.);
#6670=ORIENTED_EDGE('',*,*,#5109,.F.);
#6671=ORIENTED_EDGE('',*,*,#5119,.F.);
#6672=ORIENTED_EDGE('',*,*,#5090,.T.);
#6673=ORIENTED_EDGE('',*,*,#5118,.T.);
#6674=ORIENTED_EDGE('',*,*,#5094,.F.);
#6675=ORIENTED_EDGE('',*,*,#5120,.F.);
#6676=ORIENTED_EDGE('',*,*,#5088,.T.);
#6677=ORIENTED_EDGE('',*,*,#5119,.T.);
#6678=ORIENTED_EDGE('',*,*,#5097,.F.);
#6679=ORIENTED_EDGE('',*,*,#5121,.F.);
#6680=ORIENTED_EDGE('',*,*,#5081,.T.);
#6681=ORIENTED_EDGE('',*,*,#5120,.T.);
#6682=ORIENTED_EDGE('',*,*,#5084,.F.);
#6683=ORIENTED_EDGE('',*,*,#5035,.T.);
#6684=ORIENTED_EDGE('',*,*,#5041,.F.);
#6685=ORIENTED_EDGE('',*,*,#5053,.F.);
#6686=ORIENTED_EDGE('',*,*,#5079,.T.);
#6687=ORIENTED_EDGE('',*,*,#5121,.T.);
#6688=ORIENTED_EDGE('',*,*,#5074,.F.);
#6689=ORIENTED_EDGE('',*,*,#5122,.F.);
#6690=ORIENTED_EDGE('',*,*,#5071,.T.);
#6691=ORIENTED_EDGE('',*,*,#5051,.T.);
#6692=ORIENTED_EDGE('',*,*,#5043,.T.);
#6693=ORIENTED_EDGE('',*,*,#5037,.T.);
#6694=ORIENTED_EDGE('',*,*,#5076,.F.);
#6695=ORIENTED_EDGE('',*,*,#5123,.F.);
#6696=ORIENTED_EDGE('',*,*,#5061,.T.);
#6697=ORIENTED_EDGE('',*,*,#5122,.T.);
#6698=ORIENTED_EDGE('',*,*,#5065,.F.);
#6699=ORIENTED_EDGE('',*,*,#5124,.F.);
#6700=ORIENTED_EDGE('',*,*,#5058,.T.);
#6701=ORIENTED_EDGE('',*,*,#5123,.T.);
#6702=ORIENTED_EDGE('',*,*,#5068,.F.);
#6703=ORIENTED_EDGE('',*,*,#5125,.F.);
#6704=ORIENTED_EDGE('',*,*,#5126,.T.);
#6705=ORIENTED_EDGE('',*,*,#5124,.T.);
#6706=ORIENTED_EDGE('',*,*,#5029,.F.);
#6707=ORIENTED_EDGE('',*,*,#5032,.F.);
#6708=ORIENTED_EDGE('',*,*,#5070,.F.);
#6709=ORIENTED_EDGE('',*,*,#5127,.F.);
#6710=ORIENTED_EDGE('',*,*,#5128,.T.);
#6711=ORIENTED_EDGE('',*,*,#5125,.T.);
#6712=ORIENTED_EDGE('',*,*,#5069,.T.);
#6713=ORIENTED_EDGE('',*,*,#5129,.F.);
#6714=ORIENTED_EDGE('',*,*,#5130,.F.);
#6715=ORIENTED_EDGE('',*,*,#5127,.T.);
#6716=ORIENTED_EDGE('',*,*,#5027,.T.);
#6717=ORIENTED_EDGE('',*,*,#5030,.T.);
#6718=ORIENTED_EDGE('',*,*,#5067,.T.);
#6719=ORIENTED_EDGE('',*,*,#5131,.F.);
#6720=ORIENTED_EDGE('',*,*,#5060,.F.);
#6721=ORIENTED_EDGE('',*,*,#5129,.T.);
#6722=ORIENTED_EDGE('',*,*,#5077,.T.);
#6723=ORIENTED_EDGE('',*,*,#5132,.F.);
#6724=ORIENTED_EDGE('',*,*,#5062,.F.);
#6725=ORIENTED_EDGE('',*,*,#5131,.T.);
#6726=ORIENTED_EDGE('',*,*,#5075,.T.);
#6727=ORIENTED_EDGE('',*,*,#5039,.F.);
#6728=ORIENTED_EDGE('',*,*,#5133,.F.);
#6729=ORIENTED_EDGE('',*,*,#5048,.F.);
#6730=ORIENTED_EDGE('',*,*,#5134,.F.);
#6731=ORIENTED_EDGE('',*,*,#5049,.F.);
#6732=ORIENTED_EDGE('',*,*,#5072,.F.);
#6733=ORIENTED_EDGE('',*,*,#5132,.T.);
#6734=ORIENTED_EDGE('',*,*,#5086,.T.);
#6735=ORIENTED_EDGE('',*,*,#5135,.F.);
#6736=ORIENTED_EDGE('',*,*,#5080,.F.);
#6737=ORIENTED_EDGE('',*,*,#5055,.T.);
#6738=ORIENTED_EDGE('',*,*,#5136,.T.);
#6739=ORIENTED_EDGE('',*,*,#5046,.T.);
#6740=ORIENTED_EDGE('',*,*,#5137,.F.);
#6741=ORIENTED_EDGE('',*,*,#5033,.F.);
#6742=ORIENTED_EDGE('',*,*,#5098,.T.);
#6743=ORIENTED_EDGE('',*,*,#5138,.F.);
#6744=ORIENTED_EDGE('',*,*,#5082,.F.);
#6745=ORIENTED_EDGE('',*,*,#5135,.T.);
#6746=ORIENTED_EDGE('',*,*,#5096,.T.);
#6747=ORIENTED_EDGE('',*,*,#5139,.F.);
#6748=ORIENTED_EDGE('',*,*,#5089,.F.);
#6749=ORIENTED_EDGE('',*,*,#5138,.T.);
#6750=ORIENTED_EDGE('',*,*,#5110,.T.);
#6751=ORIENTED_EDGE('',*,*,#5140,.F.);
#6752=ORIENTED_EDGE('',*,*,#5091,.F.);
#6753=ORIENTED_EDGE('',*,*,#5139,.T.);
#6754=ORIENTED_EDGE('',*,*,#5108,.T.);
#6755=ORIENTED_EDGE('',*,*,#5113,.F.);
#6756=ORIENTED_EDGE('',*,*,#5101,.F.);
#6757=ORIENTED_EDGE('',*,*,#5140,.T.);
#6758=ORIENTED_EDGE('',*,*,#5130,.T.);
#6759=ORIENTED_EDGE('',*,*,#5059,.T.);
#6760=ORIENTED_EDGE('',*,*,#5126,.F.);
#6761=ORIENTED_EDGE('',*,*,#5128,.F.);
#6762=ORIENTED_EDGE('',*,*,#5111,.F.);
#6763=ORIENTED_EDGE('',*,*,#5107,.T.);
#6764=ORIENTED_EDGE('',*,*,#5116,.T.);
#6765=ORIENTED_EDGE('',*,*,#5114,.T.);
#6766=ORIENTED_EDGE('',*,*,#5136,.F.);
#6767=ORIENTED_EDGE('',*,*,#5141,.T.);
#6768=ORIENTED_EDGE('',*,*,#5142,.F.);
#6769=ORIENTED_EDGE('',*,*,#5143,.F.);
#6770=ORIENTED_EDGE('',*,*,#5144,.T.);
#6771=ORIENTED_EDGE('',*,*,#5134,.T.);
#6772=ORIENTED_EDGE('',*,*,#5145,.F.);
#6773=ORIENTED_EDGE('',*,*,#5146,.T.);
#6774=ORIENTED_EDGE('',*,*,#5044,.F.);
#6775=ORIENTED_EDGE('',*,*,#5050,.F.);
#6776=ORIENTED_EDGE('',*,*,#5144,.F.);
#6777=ORIENTED_EDGE('',*,*,#5147,.T.);
#6778=ORIENTED_EDGE('',*,*,#5141,.F.);
#6779=ORIENTED_EDGE('',*,*,#5054,.F.);
#6780=ORIENTED_EDGE('',*,*,#5047,.T.);
#6781=ORIENTED_EDGE('',*,*,#5143,.T.);
#6782=ORIENTED_EDGE('',*,*,#5148,.T.);
#6783=ORIENTED_EDGE('',*,*,#5145,.T.);
#6784=ORIENTED_EDGE('',*,*,#5146,.F.);
#6785=ORIENTED_EDGE('',*,*,#5149,.T.);
#6786=ORIENTED_EDGE('',*,*,#5150,.F.);
#6787=ORIENTED_EDGE('',*,*,#5151,.F.);
#6788=ORIENTED_EDGE('',*,*,#5152,.F.);
#6789=ORIENTED_EDGE('',*,*,#5153,.F.);
#6790=ORIENTED_EDGE('',*,*,#5154,.T.);
#6791=ORIENTED_EDGE('',*,*,#5142,.T.);
#6792=ORIENTED_EDGE('',*,*,#5147,.F.);
#6793=ORIENTED_EDGE('',*,*,#5151,.T.);
#6794=ORIENTED_EDGE('',*,*,#5155,.T.);
#6795=ORIENTED_EDGE('',*,*,#5156,.T.);
#6796=ORIENTED_EDGE('',*,*,#5157,.T.);
#6797=ORIENTED_EDGE('',*,*,#5152,.T.);
#6798=ORIENTED_EDGE('',*,*,#5011,.F.);
#6799=ORIENTED_EDGE('',*,*,#5014,.F.);
#6800=ORIENTED_EDGE('',*,*,#5149,.F.);
#6801=ORIENTED_EDGE('',*,*,#5148,.F.);
#6802=ORIENTED_EDGE('',*,*,#5154,.F.);
#6803=ORIENTED_EDGE('',*,*,#5158,.F.);
#6804=ORIENTED_EDGE('',*,*,#5159,.F.);
#6805=ORIENTED_EDGE('',*,*,#5160,.F.);
#6806=ORIENTED_EDGE('',*,*,#5009,.F.);
#6807=ORIENTED_EDGE('',*,*,#5012,.F.);
#6808=ORIENTED_EDGE('',*,*,#5160,.T.);
#6809=ORIENTED_EDGE('',*,*,#5161,.T.);
#6810=ORIENTED_EDGE('',*,*,#5155,.F.);
#6811=ORIENTED_EDGE('',*,*,#5150,.T.);
#6812=ORIENTED_EDGE('',*,*,#5157,.F.);
#6813=ORIENTED_EDGE('',*,*,#5162,.F.);
#6814=ORIENTED_EDGE('',*,*,#5158,.T.);
#6815=ORIENTED_EDGE('',*,*,#5153,.T.);
#6816=ORIENTED_EDGE('',*,*,#5156,.F.);
#6817=ORIENTED_EDGE('',*,*,#5161,.F.);
#6818=ORIENTED_EDGE('',*,*,#5159,.T.);
#6819=ORIENTED_EDGE('',*,*,#5162,.T.);
#6820=ORIENTED_EDGE('',*,*,#5163,.F.);
#6821=ORIENTED_EDGE('',*,*,#5133,.T.);
#6822=ORIENTED_EDGE('',*,*,#5164,.T.);
#6823=ORIENTED_EDGE('',*,*,#5165,.F.);
#6824=ORIENTED_EDGE('',*,*,#5166,.T.);
#6825=ORIENTED_EDGE('',*,*,#5137,.T.);
#6826=ORIENTED_EDGE('',*,*,#5167,.F.);
#6827=ORIENTED_EDGE('',*,*,#5168,.T.);
#6828=ORIENTED_EDGE('',*,*,#5042,.F.);
#6829=ORIENTED_EDGE('',*,*,#5034,.F.);
#6830=ORIENTED_EDGE('',*,*,#5166,.F.);
#6831=ORIENTED_EDGE('',*,*,#5169,.T.);
#6832=ORIENTED_EDGE('',*,*,#5164,.F.);
#6833=ORIENTED_EDGE('',*,*,#5038,.F.);
#6834=ORIENTED_EDGE('',*,*,#5045,.T.);
#6835=ORIENTED_EDGE('',*,*,#5163,.T.);
#6836=ORIENTED_EDGE('',*,*,#5170,.T.);
#6837=ORIENTED_EDGE('',*,*,#5167,.T.);
#6838=ORIENTED_EDGE('',*,*,#5165,.T.);
#6839=ORIENTED_EDGE('',*,*,#5171,.F.);
#6840=ORIENTED_EDGE('',*,*,#5172,.T.);
#6841=ORIENTED_EDGE('',*,*,#5173,.T.);
#6842=ORIENTED_EDGE('',*,*,#5174,.T.);
#6843=ORIENTED_EDGE('',*,*,#5175,.T.);
#6844=ORIENTED_EDGE('',*,*,#5176,.F.);
#6845=ORIENTED_EDGE('',*,*,#5168,.F.);
#6846=ORIENTED_EDGE('',*,*,#5169,.F.);
#6847=ORIENTED_EDGE('',*,*,#5176,.T.);
#6848=ORIENTED_EDGE('',*,*,#5177,.T.);
#6849=ORIENTED_EDGE('',*,*,#5178,.T.);
#6850=ORIENTED_EDGE('',*,*,#5179,.T.);
#6851=ORIENTED_EDGE('',*,*,#5171,.T.);
#6852=ORIENTED_EDGE('',*,*,#5015,.T.);
#6853=ORIENTED_EDGE('',*,*,#5018,.T.);
#6854=ORIENTED_EDGE('',*,*,#5174,.F.);
#6855=ORIENTED_EDGE('',*,*,#5170,.F.);
#6856=ORIENTED_EDGE('',*,*,#5173,.F.);
#6857=ORIENTED_EDGE('',*,*,#5180,.F.);
#6858=ORIENTED_EDGE('',*,*,#5181,.F.);
#6859=ORIENTED_EDGE('',*,*,#5182,.F.);
#6860=ORIENTED_EDGE('',*,*,#5017,.F.);
#6861=ORIENTED_EDGE('',*,*,#5020,.F.);
#6862=ORIENTED_EDGE('',*,*,#5180,.T.);
#6863=ORIENTED_EDGE('',*,*,#5172,.F.);
#6864=ORIENTED_EDGE('',*,*,#5179,.F.);
#6865=ORIENTED_EDGE('',*,*,#5183,.F.);
#6866=ORIENTED_EDGE('',*,*,#5178,.F.);
#6867=ORIENTED_EDGE('',*,*,#5184,.F.);
#6868=ORIENTED_EDGE('',*,*,#5181,.T.);
#6869=ORIENTED_EDGE('',*,*,#5183,.T.);
#6870=ORIENTED_EDGE('',*,*,#5177,.F.);
#6871=ORIENTED_EDGE('',*,*,#5175,.F.);
#6872=ORIENTED_EDGE('',*,*,#5182,.T.);
#6873=ORIENTED_EDGE('',*,*,#5184,.T.);
#8833=CYLINDRICAL_SURFACE('',#9887,6.00000000000001);
#8834=CYLINDRICAL_SURFACE('',#9890,6.00000000000001);
#8835=CYLINDRICAL_SURFACE('',#9893,6.00000000000001);
#8836=CYLINDRICAL_SURFACE('',#9896,6.00000000000001);
#8837=CYLINDRICAL_SURFACE('',#9899,6.34999999999994);
#8838=CYLINDRICAL_SURFACE('',#9902,6.34999999999997);
#8839=CYLINDRICAL_SURFACE('',#9905,6.34999999999995);
#8840=CYLINDRICAL_SURFACE('',#9908,6.34999999999997);
#8841=CYLINDRICAL_SURFACE('',#9962,4.);
#8842=CYLINDRICAL_SURFACE('',#9964,4.);
#8843=CYLINDRICAL_SURFACE('',#9966,4.);
#8844=CYLINDRICAL_SURFACE('',#9967,4.);
#8845=CYLINDRICAL_SURFACE('',#9969,4.);
#8846=CYLINDRICAL_SURFACE('',#9973,1.);
#8847=CYLINDRICAL_SURFACE('',#9975,1.);
#8848=CYLINDRICAL_SURFACE('',#9976,1.);
#8849=CYLINDRICAL_SURFACE('',#9978,1.);
#8850=CYLINDRICAL_SURFACE('',#9980,1.);
#8851=CYLINDRICAL_SURFACE('',#9989,4.);
#8852=CYLINDRICAL_SURFACE('',#9990,1.);
#8853=CYLINDRICAL_SURFACE('',#10004,4.);
#8854=CYLINDRICAL_SURFACE('',#10005,1.);
#9061=ADVANCED_FACE('',(#922),#8833,.F.);
#9062=ADVANCED_FACE('',(#923),#8834,.F.);
#9063=ADVANCED_FACE('',(#924),#8835,.F.);
#9064=ADVANCED_FACE('',(#925),#8836,.F.);
#9065=ADVANCED_FACE('',(#926),#8837,.F.);
#9066=ADVANCED_FACE('',(#927),#8838,.F.);
#9067=ADVANCED_FACE('',(#928),#8839,.F.);
#9068=ADVANCED_FACE('',(#929),#8840,.F.);
#9069=ADVANCED_FACE('',(#930),#558,.T.);
#9070=ADVANCED_FACE('',(#931),#559,.T.);
#9071=ADVANCED_FACE('',(#932),#560,.T.);
#9072=ADVANCED_FACE('',(#933),#561,.F.);
#9073=ADVANCED_FACE('',(#934),#562,.T.);
#9074=ADVANCED_FACE('',(#935),#563,.T.);
#9075=ADVANCED_FACE('',(#936),#564,.T.);
#9076=ADVANCED_FACE('',(#937),#565,.T.);
#9077=ADVANCED_FACE('',(#938),#566,.T.);
#9078=ADVANCED_FACE('',(#939),#567,.T.);
#9079=ADVANCED_FACE('',(#940),#568,.T.);
#9080=ADVANCED_FACE('',(#941),#569,.T.);
#9081=ADVANCED_FACE('',(#942),#570,.T.);
#9082=ADVANCED_FACE('',(#943),#571,.T.);
#9083=ADVANCED_FACE('',(#944),#572,.T.);
#9084=ADVANCED_FACE('',(#945),#573,.T.);
#9085=ADVANCED_FACE('',(#946),#574,.T.);
#9086=ADVANCED_FACE('',(#947),#575,.T.);
#9087=ADVANCED_FACE('',(#948),#576,.T.);
#9088=ADVANCED_FACE('',(#949),#577,.T.);
#9089=ADVANCED_FACE('',(#950),#578,.T.);
#9090=ADVANCED_FACE('',(#951),#579,.T.);
#9091=ADVANCED_FACE('',(#952),#580,.T.);
#9092=ADVANCED_FACE('',(#953),#581,.T.);
#9093=ADVANCED_FACE('',(#954,#401,#402),#582,.F.);
#9094=ADVANCED_FACE('',(#955),#583,.T.);
#9095=ADVANCED_FACE('',(#956,#403,#404),#584,.T.);
#9096=ADVANCED_FACE('',(#957),#8841,.T.);
#9097=ADVANCED_FACE('',(#958),#585,.T.);
#9098=ADVANCED_FACE('',(#959),#8842,.T.);
#9099=ADVANCED_FACE('',(#960),#586,.T.);
#9100=ADVANCED_FACE('',(#961),#8843,.T.);
#9101=ADVANCED_FACE('',(#962),#8844,.T.);
#9102=ADVANCED_FACE('',(#963),#587,.T.);
#9103=ADVANCED_FACE('',(#964),#8845,.T.);
#9104=ADVANCED_FACE('',(#965,#405,#406),#588,.T.);
#9105=ADVANCED_FACE('',(#966),#589,.T.);
#9106=ADVANCED_FACE('',(#967,#407,#408),#590,.F.);
#9107=ADVANCED_FACE('',(#968),#8846,.F.);
#9108=ADVANCED_FACE('',(#969),#591,.F.);
#9109=ADVANCED_FACE('',(#970),#8847,.F.);
#9110=ADVANCED_FACE('',(#971),#8848,.F.);
#9111=ADVANCED_FACE('',(#972),#592,.F.);
#9112=ADVANCED_FACE('',(#973),#8849,.F.);
#9113=ADVANCED_FACE('',(#974),#593,.F.);
#9114=ADVANCED_FACE('',(#975),#8850,.F.);
#9115=ADVANCED_FACE('',(#976),#594,.T.);
#9116=ADVANCED_FACE('',(#977),#595,.F.);
#9117=ADVANCED_FACE('',(#978),#596,.T.);
#9118=ADVANCED_FACE('',(#979),#597,.F.);
#9119=ADVANCED_FACE('',(#980),#8851,.T.);
#9120=ADVANCED_FACE('',(#981),#8852,.F.);
#9121=ADVANCED_FACE('',(#982),#598,.F.);
#9122=ADVANCED_FACE('',(#983),#599,.F.);
#9123=ADVANCED_FACE('',(#984,#409,#410),#600,.F.);
#9124=ADVANCED_FACE('',(#985,#411,#412),#601,.T.);
#9125=ADVANCED_FACE('',(#986),#602,.F.);
#9126=ADVANCED_FACE('',(#987),#603,.T.);
#9127=ADVANCED_FACE('',(#988),#604,.T.);
#9128=ADVANCED_FACE('',(#989),#605,.T.);
#9129=ADVANCED_FACE('',(#990),#606,.F.);
#9130=ADVANCED_FACE('',(#991),#8853,.T.);
#9131=ADVANCED_FACE('',(#992),#8854,.F.);
#9132=ADVANCED_FACE('',(#993),#607,.F.);
#9133=ADVANCED_FACE('',(#994),#608,.F.);
#9134=ADVANCED_FACE('',(#995,#413,#414),#609,.F.);
#9135=ADVANCED_FACE('',(#996,#415,#416),#610,.T.);
#9136=ADVANCED_FACE('',(#997),#611,.F.);
#9137=ADVANCED_FACE('',(#998),#612,.T.);
#9138=ADVANCED_FACE('',(#999),#613,.T.);
#9557=CLOSED_SHELL('',(#9061,#9062,#9063,#9064,#9065,#9066,#9067,#9068,
#9069,#9070,#9071,#9072,#9073,#9074,#9075,#9076,#9077,#9078,#9079,#9080,
#9081,#9082,#9083,#9084,#9085,#9086,#9087,#9088,#9089,#9090,#9091,#9092,
#9093,#9094,#9095,#9096,#9097,#9098,#9099,#9100,#9101,#9102,#9103,#9104,
#9105,#9106,#9107,#9108,#9109,#9110,#9111,#9112,#9113,#9114,#9115,#9116,
#9117,#9118,#9119,#9120,#9121,#9122,#9123,#9124,#9125,#9126,#9127,#9128,
#9129,#9130,#9131,#9132,#9133,#9134,#9135,#9136,#9137,#9138));
#9886=AXIS2_PLACEMENT_3D('',#14183,#11266,#11267);
#9887=AXIS2_PLACEMENT_3D('',#14184,#11268,#11269);
#9888=AXIS2_PLACEMENT_3D('',#14186,#11270,#11271);
#9889=AXIS2_PLACEMENT_3D('',#14189,#11273,#11274);
#9890=AXIS2_PLACEMENT_3D('',#14190,#11275,#11276);
#9891=AXIS2_PLACEMENT_3D('',#14192,#11277,#11278);
#9892=AXIS2_PLACEMENT_3D('',#14195,#11280,#11281);
#9893=AXIS2_PLACEMENT_3D('',#14196,#11282,#11283);
#9894=AXIS2_PLACEMENT_3D('',#14198,#11284,#11285);
#9895=AXIS2_PLACEMENT_3D('',#14201,#11287,#11288);
#9896=AXIS2_PLACEMENT_3D('',#14202,#11289,#11290);
#9897=AXIS2_PLACEMENT_3D('',#14204,#11291,#11292);
#9898=AXIS2_PLACEMENT_3D('',#14207,#11294,#11295);
#9899=AXIS2_PLACEMENT_3D('',#14208,#11296,#11297);
#9900=AXIS2_PLACEMENT_3D('',#14210,#11298,#11299);
#9901=AXIS2_PLACEMENT_3D('',#14213,#11301,#11302);
#9902=AXIS2_PLACEMENT_3D('',#14214,#11303,#11304);
#9903=AXIS2_PLACEMENT_3D('',#14216,#11305,#11306);
#9904=AXIS2_PLACEMENT_3D('',#14219,#11308,#11309);
#9905=AXIS2_PLACEMENT_3D('',#14220,#11310,#11311);
#9906=AXIS2_PLACEMENT_3D('',#14222,#11312,#11313);
#9907=AXIS2_PLACEMENT_3D('',#14225,#11315,#11316);
#9908=AXIS2_PLACEMENT_3D('',#14226,#11317,#11318);
#9909=AXIS2_PLACEMENT_3D('',#14228,#11319,#11320);
#9910=AXIS2_PLACEMENT_3D('',#14231,#11322,#11323);
#9911=AXIS2_PLACEMENT_3D('',#14232,#11324,#11325);
#9912=AXIS2_PLACEMENT_3D('',#14237,#11327,#11328);
#9913=AXIS2_PLACEMENT_3D('',#14241,#11331,#11332);
#9914=AXIS2_PLACEMENT_3D('',#14246,#11334,#11335);
#9915=AXIS2_PLACEMENT_3D('',#14250,#11338,#11339);
#9916=AXIS2_PLACEMENT_3D('',#14257,#11344,#11345);
#9917=AXIS2_PLACEMENT_3D('',#14266,#11350,#11351);
#9918=AXIS2_PLACEMENT_3D('',#14270,#11353,#11354);
#9919=AXIS2_PLACEMENT_3D('',#14274,#11357,#11358);
#9920=AXIS2_PLACEMENT_3D('',#14278,#11360,#11361);
#9921=AXIS2_PLACEMENT_3D('',#14282,#11364,#11365);
#9922=AXIS2_PLACEMENT_3D('',#14287,#11367,#11368);
#9923=AXIS2_PLACEMENT_3D('',#14290,#11370,#11371);
#9924=AXIS2_PLACEMENT_3D('',#14291,#11372,#11373);
#9925=AXIS2_PLACEMENT_3D('',#14297,#11377,#11378);
#9926=AXIS2_PLACEMENT_3D('',#14302,#11380,#11381);
#9927=AXIS2_PLACEMENT_3D('',#14305,#11383,#11384);
#9928=AXIS2_PLACEMENT_3D('',#14306,#11385,#11386);
#9929=AXIS2_PLACEMENT_3D('',#14312,#11390,#11391);
#9930=AXIS2_PLACEMENT_3D('',#14313,#11392,#11393);
#9931=AXIS2_PLACEMENT_3D('',#14314,#11394,#11395);
#9932=AXIS2_PLACEMENT_3D('',#14315,#11396,#11397);
#9933=AXIS2_PLACEMENT_3D('',#14319,#11399,#11400);
#9934=AXIS2_PLACEMENT_3D('',#14320,#11401,#11402);
#9935=AXIS2_PLACEMENT_3D('',#14321,#11403,#11404);
#9936=AXIS2_PLACEMENT_3D('',#14324,#11407,#11408);
#9937=AXIS2_PLACEMENT_3D('',#14328,#11410,#11411);
#9938=AXIS2_PLACEMENT_3D('',#14329,#11412,#11413);
#9939=AXIS2_PLACEMENT_3D('',#14330,#11414,#11415);
#9940=AXIS2_PLACEMENT_3D('',#14336,#11419,#11420);
#9941=AXIS2_PLACEMENT_3D('',#14338,#11421,#11422);
#9942=AXIS2_PLACEMENT_3D('',#14341,#11424,#11425);
#9943=AXIS2_PLACEMENT_3D('',#14342,#11426,#11427);
#9944=AXIS2_PLACEMENT_3D('',#14346,#11429,#11430);
#9945=AXIS2_PLACEMENT_3D('',#14347,#11431,#11432);
#9946=AXIS2_PLACEMENT_3D('',#14348,#11433,#11434);
#9947=AXIS2_PLACEMENT_3D('',#14354,#11438,#11439);
#9948=AXIS2_PLACEMENT_3D('',#14359,#11441,#11442);
#9949=AXIS2_PLACEMENT_3D('',#14362,#11444,#11445);
#9950=AXIS2_PLACEMENT_3D('',#14363,#11446,#11447);
#9951=AXIS2_PLACEMENT_3D('',#14366,#11450,#11451);
#9952=AXIS2_PLACEMENT_3D('',#14370,#11453,#11454);
#9953=AXIS2_PLACEMENT_3D('',#14371,#11455,#11456);
#9954=AXIS2_PLACEMENT_3D('',#14372,#11457,#11458);
#9955=AXIS2_PLACEMENT_3D('',#14378,#11462,#11463);
#9956=AXIS2_PLACEMENT_3D('',#14383,#11465,#11466);
#9957=AXIS2_PLACEMENT_3D('',#14386,#11468,#11469);
#9958=AXIS2_PLACEMENT_3D('',#14387,#11470,#11471);
#9959=AXIS2_PLACEMENT_3D('',#14390,#11474,#11475);
#9960=AXIS2_PLACEMENT_3D('',#14395,#11479,#11480);
#9961=AXIS2_PLACEMENT_3D('',#14399,#11483,#11484);
#9962=AXIS2_PLACEMENT_3D('',#14402,#11487,#11488);
#9963=AXIS2_PLACEMENT_3D('',#14404,#11490,#11491);
#9964=AXIS2_PLACEMENT_3D('',#14406,#11493,#11494);
#9965=AXIS2_PLACEMENT_3D('',#14408,#11496,#11497);
#9966=AXIS2_PLACEMENT_3D('',#14410,#11499,#11500);
#9967=AXIS2_PLACEMENT_3D('',#14411,#11501,#11502);
#9968=AXIS2_PLACEMENT_3D('',#14413,#11504,#11505);
#9969=AXIS2_PLACEMENT_3D('',#14415,#11507,#11508);
#9970=AXIS2_PLACEMENT_3D('',#14417,#11510,#11511);
#9971=AXIS2_PLACEMENT_3D('',#14421,#11514,#11515);
#9972=AXIS2_PLACEMENT_3D('',#14425,#11518,#11519);
#9973=AXIS2_PLACEMENT_3D('',#14428,#11522,#11523);
#9974=AXIS2_PLACEMENT_3D('',#14430,#11525,#11526);
#9975=AXIS2_PLACEMENT_3D('',#14432,#11528,#11529);
#9976=AXIS2_PLACEMENT_3D('',#14435,#11532,#11533);
#9977=AXIS2_PLACEMENT_3D('',#14439,#11537,#11538);
#9978=AXIS2_PLACEMENT_3D('',#14441,#11540,#11541);
#9979=AXIS2_PLACEMENT_3D('',#14443,#11543,#11544);
#9980=AXIS2_PLACEMENT_3D('',#14445,#11546,#11547);
#9981=AXIS2_PLACEMENT_3D('',#14446,#11548,#11549);
#9982=AXIS2_PLACEMENT_3D('',#14447,#11550,#11551);
#9983=AXIS2_PLACEMENT_3D('',#14448,#11552,#11553);
#9984=AXIS2_PLACEMENT_3D('',#14450,#11554,#11555);
#9985=AXIS2_PLACEMENT_3D('',#14453,#11557,#11558);
#9986=AXIS2_PLACEMENT_3D('',#14454,#11559,#11560);
#9987=AXIS2_PLACEMENT_3D('',#14456,#11561,#11562);
#9988=AXIS2_PLACEMENT_3D('',#14458,#11563,#11564);
#9989=AXIS2_PLACEMENT_3D('',#14460,#11566,#11567);
#9990=AXIS2_PLACEMENT_3D('',#14462,#11569,#11570);
#9991=AXIS2_PLACEMENT_3D('',#14464,#11572,#11573);
#9992=AXIS2_PLACEMENT_3D('',#14470,#11577,#11578);
#9993=AXIS2_PLACEMENT_3D('',#14476,#11582,#11583);
#9994=AXIS2_PLACEMENT_3D('',#14482,#11587,#11588);
#9995=AXIS2_PLACEMENT_3D('',#14488,#11592,#11593);
#9996=AXIS2_PLACEMENT_3D('',#14490,#11595,#11596);
#9997=AXIS2_PLACEMENT_3D('',#14492,#11598,#11599);
#9998=AXIS2_PLACEMENT_3D('',#14493,#11600,#11601);
#9999=AXIS2_PLACEMENT_3D('',#14495,#11602,#11603);
#10000=AXIS2_PLACEMENT_3D('',#14497,#11604,#11605);
#10001=AXIS2_PLACEMENT_3D('',#14499,#11607,#11608);
#10002=AXIS2_PLACEMENT_3D('',#14501,#11609,#11610);
#10003=AXIS2_PLACEMENT_3D('',#14503,#11611,#11612);
#10004=AXIS2_PLACEMENT_3D('',#14505,#11614,#11615);
#10005=AXIS2_PLACEMENT_3D('',#14507,#11617,#11618);
#10006=AXIS2_PLACEMENT_3D('',#14509,#11620,#11621);
#10007=AXIS2_PLACEMENT_3D('',#14515,#11625,#11626);
#10008=AXIS2_PLACEMENT_3D('',#14521,#11630,#11631);
#10009=AXIS2_PLACEMENT_3D('',#14527,#11635,#11636);
#10010=AXIS2_PLACEMENT_3D('',#14533,#11640,#11641);
#10011=AXIS2_PLACEMENT_3D('',#14535,#11643,#11644);
#10012=AXIS2_PLACEMENT_3D('',#14537,#11646,#11647);
#11266=DIRECTION('axis',(0.,0.,1.));
#11267=DIRECTION('refdir',(1.,0.,0.));
#11268=DIRECTION('center_axis',(0.,0.,1.));
#11269=DIRECTION('ref_axis',(1.,0.,0.));
#11270=DIRECTION('center_axis',(0.,-3.89551938464967E-15,-1.));
#11271=DIRECTION('ref_axis',(0.,1.,-3.89551938464967E-15));
#11272=DIRECTION('',(0.,0.,1.));
#11273=DIRECTION('center_axis',(0.,0.,1.));
#11274=DIRECTION('ref_axis',(1.,0.,0.));
#11275=DIRECTION('center_axis',(0.,0.,1.));
#11276=DIRECTION('ref_axis',(1.,0.,0.));
#11277=DIRECTION('center_axis',(0.,-3.89551938464967E-15,-1.));
#11278=DIRECTION('ref_axis',(0.,1.,-3.89551938464967E-15));
#11279=DIRECTION('',(0.,0.,1.));
#11280=DIRECTION('center_axis',(0.,0.,1.));
#11281=DIRECTION('ref_axis',(1.,0.,0.));
#11282=DIRECTION('center_axis',(0.,0.,1.));
#11283=DIRECTION('ref_axis',(1.,0.,0.));
#11284=DIRECTION('center_axis',(0.,0.,1.));
#11285=DIRECTION('ref_axis',(1.,0.,0.));
#11286=DIRECTION('',(0.,0.,1.));
#11287=DIRECTION('center_axis',(0.,-3.49148133884313E-15,1.));
#11288=DIRECTION('ref_axis',(0.,-1.,-3.49148133884313E-15));
#11289=DIRECTION('center_axis',(0.,0.,1.));
#11290=DIRECTION('ref_axis',(1.,0.,0.));
#11291=DIRECTION('center_axis',(0.,0.,1.));
#11292=DIRECTION('ref_axis',(1.,0.,0.));
#11293=DIRECTION('',(0.,0.,1.));
#11294=DIRECTION('center_axis',(0.,-3.49148133884313E-15,1.));
#11295=DIRECTION('ref_axis',(0.,-1.,-3.49148133884313E-15));
#11296=DIRECTION('center_axis',(0.,-1.,0.));
#11297=DIRECTION('ref_axis',(0.,0.,-1.));
#11298=DIRECTION('center_axis',(1.22464679914735E-16,-1.,0.));
#11299=DIRECTION('ref_axis',(1.,1.22464679914735E-16,0.));
#11300=DIRECTION('',(0.,-1.,0.));
#11301=DIRECTION('center_axis',(0.,-1.,0.));
#11302=DIRECTION('ref_axis',(0.,0.,1.));
#11303=DIRECTION('center_axis',(0.,-1.,0.));
#11304=DIRECTION('ref_axis',(0.,0.,-1.));
#11305=DIRECTION('center_axis',(1.22464679914735E-16,-1.,0.));
#11306=DIRECTION('ref_axis',(1.,1.22464679914735E-16,0.));
#11307=DIRECTION('',(0.,-1.,0.));
#11308=DIRECTION('center_axis',(0.,-1.,0.));
#11309=DIRECTION('ref_axis',(0.,0.,-1.));
#11310=DIRECTION('center_axis',(0.,-1.,0.));
#11311=DIRECTION('ref_axis',(0.,0.,-1.));
#11312=DIRECTION('center_axis',(0.,-1.,0.));
#11313=DIRECTION('ref_axis',(0.,0.,-1.));
#11314=DIRECTION('',(0.,-1.,0.));
#11315=DIRECTION('center_axis',(0.,-1.,0.));
#11316=DIRECTION('ref_axis',(0.,0.,1.));
#11317=DIRECTION('center_axis',(0.,-1.,0.));
#11318=DIRECTION('ref_axis',(0.,0.,-1.));
#11319=DIRECTION('center_axis',(0.,-1.,0.));
#11320=DIRECTION('ref_axis',(0.,0.,-1.));
#11321=DIRECTION('',(0.,-1.,0.));
#11322=DIRECTION('center_axis',(0.,-1.,0.));
#11323=DIRECTION('ref_axis',(0.,0.,-1.));
#11324=DIRECTION('center_axis',(-1.,0.,0.));
#11325=DIRECTION('ref_axis',(0.,0.,1.));
#11326=DIRECTION('',(0.,0.,1.));
#11327=DIRECTION('center_axis',(1.,0.,0.));
#11328=DIRECTION('ref_axis',(0.,0.,-1.));
#11329=DIRECTION('',(0.,0.,1.));
#11330=DIRECTION('',(0.,-1.,0.));
#11331=DIRECTION('center_axis',(1.,5.31105888065192E-32,-8.67361737988404E-16));
#11332=DIRECTION('ref_axis',(-8.67361737988404E-16,0.,-1.));
#11333=DIRECTION('',(0.,0.,-1.));
#11334=DIRECTION('center_axis',(-1.,0.,0.));
#11335=DIRECTION('ref_axis',(0.,0.,-1.));
#11336=DIRECTION('',(-8.67361737988404E-16,0.,-1.));
#11337=DIRECTION('',(0.,1.,0.));
#11338=DIRECTION('center_axis',(0.,1.,0.));
#11339=DIRECTION('ref_axis',(0.,0.,1.));
#11340=DIRECTION('',(0.,0.,-1.));
#11341=DIRECTION('',(-1.,0.,0.));
#11342=DIRECTION('',(0.,0.,-1.));
#11343=DIRECTION('',(1.,0.,0.));
#11344=DIRECTION('center_axis',(0.,1.,0.));
#11345=DIRECTION('ref_axis',(0.,0.,1.));
#11346=DIRECTION('',(-1.,0.,0.));
#11347=DIRECTION('',(0.,0.,-1.));
#11348=DIRECTION('',(1.,0.,0.));
#11349=DIRECTION('',(0.,0.,-1.));
#11350=DIRECTION('center_axis',(1.,-3.98329416048893E-32,6.50521303491302E-16));
#11351=DIRECTION('ref_axis',(6.50521303491302E-16,0.,-1.));
#11352=DIRECTION('',(0.,0.,-1.));
#11353=DIRECTION('center_axis',(-1.,0.,0.));
#11354=DIRECTION('ref_axis',(0.,0.,1.));
#11355=DIRECTION('',(0.,0.,-1.));
#11356=DIRECTION('',(0.,-1.,0.));
#11357=DIRECTION('center_axis',(-1.,0.,0.));
#11358=DIRECTION('ref_axis',(0.,0.,1.));
#11359=DIRECTION('',(0.,0.,-1.));
#11360=DIRECTION('center_axis',(1.,0.,0.));
#11361=DIRECTION('ref_axis',(0.,-2.42861286636753E-14,1.));
#11362=DIRECTION('',(0.,0.,-1.));
#11363=DIRECTION('',(0.,1.,0.));
#11364=DIRECTION('center_axis',(0.,0.,1.));
#11365=DIRECTION('ref_axis',(1.,0.,0.));
#11366=DIRECTION('',(1.,0.,0.));
#11367=DIRECTION('center_axis',(0.,0.,-1.));
#11368=DIRECTION('ref_axis',(1.,0.,0.));
#11369=DIRECTION('',(0.,-1.,0.));
#11370=DIRECTION('center_axis',(0.,0.,-1.));
#11371=DIRECTION('ref_axis',(1.,0.,0.));
#11372=DIRECTION('center_axis',(0.,0.,1.));
#11373=DIRECTION('ref_axis',(1.,0.,0.));
#11374=DIRECTION('',(0.,1.,0.));
#11375=DIRECTION('',(0.,1.,0.));
#11376=DIRECTION('',(-1.,0.,0.));
#11377=DIRECTION('center_axis',(0.,0.,-1.));
#11378=DIRECTION('ref_axis',(-1.,0.,0.));
#11379=DIRECTION('',(0.,1.,0.));
#11380=DIRECTION('center_axis',(0.,0.,-1.));
#11381=DIRECTION('ref_axis',(1.,0.,0.));
#11382=DIRECTION('',(-1.,0.,0.));
#11383=DIRECTION('center_axis',(0.,0.,-1.));
#11384=DIRECTION('ref_axis',(1.,0.,0.));
#11385=DIRECTION('center_axis',(0.,0.,-1.));
#11386=DIRECTION('ref_axis',(-1.,0.,0.));
#11387=DIRECTION('',(-1.,0.,0.));
#11388=DIRECTION('',(-1.,0.,0.));
#11389=DIRECTION('',(0.,-1.,0.));
#11390=DIRECTION('center_axis',(0.,0.,1.));
#11391=DIRECTION('ref_axis',(1.,0.,0.));
#11392=DIRECTION('center_axis',(0.,0.,-1.));
#11393=DIRECTION('ref_axis',(1.,0.,0.));
#11394=DIRECTION('center_axis',(0.,0.,-1.));
#11395=DIRECTION('ref_axis',(1.,0.,0.));
#11396=DIRECTION('center_axis',(0.,0.,-1.));
#11397=DIRECTION('ref_axis',(-1.,0.,0.));
#11398=DIRECTION('',(1.,0.,0.));
#11399=DIRECTION('center_axis',(0.,0.,-1.));
#11400=DIRECTION('ref_axis',(1.,0.,0.));
#11401=DIRECTION('center_axis',(0.,0.,-1.));
#11402=DIRECTION('ref_axis',(1.,0.,0.));
#11403=DIRECTION('center_axis',(0.,0.,-1.));
#11404=DIRECTION('ref_axis',(-1.,0.,0.));
#11405=DIRECTION('',(0.,1.,0.));
#11406=DIRECTION('',(0.,1.,0.));
#11407=DIRECTION('center_axis',(0.,0.,1.));
#11408=DIRECTION('ref_axis',(1.,0.,0.));
#11409=DIRECTION('',(-0.457850135121646,-0.889029388585715,0.));
#11410=DIRECTION('center_axis',(0.,0.,-1.));
#11411=DIRECTION('ref_axis',(1.,3.46944695195361E-15,0.));
#11412=DIRECTION('center_axis',(0.,0.,-1.));
#11413=DIRECTION('ref_axis',(1.,0.,0.));
#11414=DIRECTION('center_axis',(0.,0.,1.));
#11415=DIRECTION('ref_axis',(1.,0.,0.));
#11416=DIRECTION('',(0.889029388585716,-0.457850135121644,0.));
#11417=DIRECTION('',(0.889029388585716,-0.457850135121644,0.));
#11418=DIRECTION('',(0.457850135121646,0.889029388585715,0.));
#11419=DIRECTION('center_axis',(0.,0.,-1.));
#11420=DIRECTION('ref_axis',(-1.,0.,0.));
#11421=DIRECTION('center_axis',(0.,0.,-1.));
#11422=DIRECTION('ref_axis',(1.,3.46944695195361E-15,0.));
#11423=DIRECTION('',(0.457850135121646,0.889029388585715,0.));
#11424=DIRECTION('center_axis',(0.,0.,-1.));
#11425=DIRECTION('ref_axis',(1.,0.,0.));
#11426=DIRECTION('center_axis',(0.,0.,1.));
#11427=DIRECTION('ref_axis',(1.,0.,0.));
#11428=DIRECTION('',(-1.,0.,0.));
#11429=DIRECTION('center_axis',(0.,0.,-1.));
#11430=DIRECTION('ref_axis',(1.,-3.46944695195361E-15,0.));
#11431=DIRECTION('center_axis',(0.,0.,-1.));
#11432=DIRECTION('ref_axis',(1.,0.,0.));
#11433=DIRECTION('center_axis',(0.,0.,1.));
#11434=DIRECTION('ref_axis',(1.,0.,0.));
#11435=DIRECTION('',(0.,-1.,0.));
#11436=DIRECTION('',(0.,-1.,0.));
#11437=DIRECTION('',(1.,6.64977332457776E-15,0.));
#11438=DIRECTION('center_axis',(0.,0.,-1.));
#11439=DIRECTION('ref_axis',(-1.,0.,0.));
#11440=DIRECTION('',(-0.457850135121646,-0.889029388585715,0.));
#11441=DIRECTION('center_axis',(0.,0.,-1.));
#11442=DIRECTION('ref_axis',(1.,-3.46944695195361E-15,0.));
#11443=DIRECTION('',(1.,0.,0.));
#11444=DIRECTION('center_axis',(0.,0.,-1.));
#11445=DIRECTION('ref_axis',(1.,0.,0.));
#11446=DIRECTION('center_axis',(0.,0.,-1.));
#11447=DIRECTION('ref_axis',(-1.,0.,0.));
#11448=DIRECTION('',(0.889029388585716,-0.457850135121644,0.));
#11449=DIRECTION('',(0.889029388585716,-0.457850135121644,0.));
#11450=DIRECTION('center_axis',(0.,0.,1.));
#11451=DIRECTION('ref_axis',(1.,0.,0.));
#11452=DIRECTION('',(0.,1.,0.));
#11453=DIRECTION('center_axis',(0.,0.,-1.));
#11454=DIRECTION('ref_axis',(1.,0.,0.));
#11455=DIRECTION('center_axis',(0.,0.,-1.));
#11456=DIRECTION('ref_axis',(1.,0.,0.));
#11457=DIRECTION('center_axis',(0.,0.,1.));
#11458=DIRECTION('ref_axis',(1.,0.,0.));
#11459=DIRECTION('',(-1.,-1.22464679914735E-16,0.));
#11460=DIRECTION('',(-1.,-1.22464679914735E-16,0.));
#11461=DIRECTION('',(0.,1.,0.));
#11462=DIRECTION('center_axis',(0.,0.,-1.));
#11463=DIRECTION('ref_axis',(-1.,0.,0.));
#11464=DIRECTION('',(-1.,-6.64977332457776E-15,0.));
#11465=DIRECTION('center_axis',(0.,0.,-1.));
#11466=DIRECTION('ref_axis',(1.,0.,0.));
#11467=DIRECTION('',(0.,-1.,0.));
#11468=DIRECTION('center_axis',(0.,0.,-1.));
#11469=DIRECTION('ref_axis',(1.,0.,0.));
#11470=DIRECTION('center_axis',(0.,0.,-1.));
#11471=DIRECTION('ref_axis',(-1.,0.,0.));
#11472=DIRECTION('',(0.,-1.,0.));
#11473=DIRECTION('',(0.,-1.,0.));
#11474=DIRECTION('center_axis',(1.22464679914735E-16,-1.,0.));
#11475=DIRECTION('ref_axis',(1.,1.22464679914735E-16,0.));
#11476=DIRECTION('',(-1.,-1.22464679914735E-16,0.));
#11477=DIRECTION('',(0.,0.,-1.));
#11478=DIRECTION('',(0.,0.,-1.));
#11479=DIRECTION('center_axis',(-1.,0.,0.));
#11480=DIRECTION('ref_axis',(0.,0.,1.));
#11481=DIRECTION('',(0.,1.,0.));
#11482=DIRECTION('',(0.,0.,-1.));
#11483=DIRECTION('center_axis',(1.22464679914735E-16,-1.,0.));
#11484=DIRECTION('ref_axis',(1.,1.22464679914735E-16,0.));
#11485=DIRECTION('',(-1.,-1.22464679914735E-16,0.));
#11486=DIRECTION('',(0.,0.,-1.));
#11487=DIRECTION('center_axis',(0.,0.,-1.));
#11488=DIRECTION('ref_axis',(-1.,0.,0.));
#11489=DIRECTION('',(0.,0.,-1.));
#11490=DIRECTION('center_axis',(1.,0.,0.));
#11491=DIRECTION('ref_axis',(0.,0.,-1.));
#11492=DIRECTION('',(0.,0.,-1.));
#11493=DIRECTION('center_axis',(0.,0.,-1.));
#11494=DIRECTION('ref_axis',(-1.,0.,0.));
#11495=DIRECTION('',(0.,0.,-1.));
#11496=DIRECTION('center_axis',(0.457850135121644,0.889029388585716,0.));
#11497=DIRECTION('ref_axis',(-0.889029388585716,0.457850135121644,0.));
#11498=DIRECTION('',(0.,0.,-1.));
#11499=DIRECTION('center_axis',(0.,0.,-1.));
#11500=DIRECTION('ref_axis',(-1.,0.,0.));
#11501=DIRECTION('center_axis',(0.,0.,-1.));
#11502=DIRECTION('ref_axis',(-1.,0.,0.));
#11503=DIRECTION('',(0.,0.,-1.));
#11504=DIRECTION('center_axis',(-1.,0.,0.));
#11505=DIRECTION('ref_axis',(0.,0.,1.));
#11506=DIRECTION('',(0.,0.,-1.));
#11507=DIRECTION('center_axis',(0.,0.,-1.));
#11508=DIRECTION('ref_axis',(-1.,0.,0.));
#11509=DIRECTION('',(0.,0.,-1.));
#11510=DIRECTION('center_axis',(0.,-1.,0.));
#11511=DIRECTION('ref_axis',(0.,0.,-1.));
#11512=DIRECTION('',(0.,0.,-1.));
#11513=DIRECTION('',(-1.,0.,0.));
#11514=DIRECTION('center_axis',(1.,0.,0.));
#11515=DIRECTION('ref_axis',(0.,0.,-1.));
#11516=DIRECTION('',(0.,0.,-1.));
#11517=DIRECTION('',(0.,-1.,0.));
#11518=DIRECTION('center_axis',(0.,-1.,0.));
#11519=DIRECTION('ref_axis',(0.,0.,-1.));
#11520=DIRECTION('',(0.,0.,-1.));
#11521=DIRECTION('',(-1.,0.,0.));
#11522=DIRECTION('center_axis',(0.,0.,-1.));
#11523=DIRECTION('ref_axis',(-1.,0.,0.));
#11524=DIRECTION('',(0.,0.,-1.));
#11525=DIRECTION('center_axis',(-1.,0.,0.));
#11526=DIRECTION('ref_axis',(0.,0.,1.));
#11527=DIRECTION('',(0.,0.,-1.));
#11528=DIRECTION('center_axis',(0.,0.,-1.));
#11529=DIRECTION('ref_axis',(-1.,0.,0.));
#11530=DIRECTION('',(-8.67361737988404E-16,0.,-1.));
#11531=DIRECTION('',(0.,0.,-1.));
#11532=DIRECTION('center_axis',(0.,0.,-1.));
#11533=DIRECTION('ref_axis',(-1.,0.,0.));
#11534=DIRECTION('',(0.,0.,-1.));
#11535=DIRECTION('',(0.,0.,-1.));
#11536=DIRECTION('',(0.,0.,1.));
#11537=DIRECTION('center_axis',(0.457850135121644,0.889029388585716,0.));
#11538=DIRECTION('ref_axis',(-0.889029388585716,0.457850135121644,0.));
#11539=DIRECTION('',(0.,0.,-1.));
#11540=DIRECTION('center_axis',(0.,0.,-1.));
#11541=DIRECTION('ref_axis',(-1.,0.,0.));
#11542=DIRECTION('',(0.,0.,-1.));
#11543=DIRECTION('center_axis',(1.,0.,0.));
#11544=DIRECTION('ref_axis',(0.,0.,-1.));
#11545=DIRECTION('',(0.,0.,-1.));
#11546=DIRECTION('center_axis',(0.,0.,-1.));
#11547=DIRECTION('ref_axis',(-1.,0.,0.));
#11548=DIRECTION('center_axis',(0.,0.,1.));
#11549=DIRECTION('ref_axis',(1.,0.,0.));
#11550=DIRECTION('center_axis',(0.,0.,1.));
#11551=DIRECTION('ref_axis',(1.,0.,0.));
#11552=DIRECTION('center_axis',(1.,0.,0.));
#11553=DIRECTION('ref_axis',(0.,0.,-1.));
#11554=DIRECTION('center_axis',(1.,0.,0.));
#11555=DIRECTION('ref_axis',(0.,1.76941794549634E-13,1.));
#11556=DIRECTION('',(0.,0.,1.));
#11557=DIRECTION('center_axis',(1.,0.,0.));
#11558=DIRECTION('ref_axis',(0.,0.,1.));
#11559=DIRECTION('center_axis',(1.,0.,0.));
#11560=DIRECTION('ref_axis',(0.,0.,-1.));
#11561=DIRECTION('center_axis',(-1.,0.,0.));
#11562=DIRECTION('ref_axis',(0.,0.,1.));
#11563=DIRECTION('center_axis',(-1.,0.,0.));
#11564=DIRECTION('ref_axis',(0.,0.,1.));
#11565=DIRECTION('',(0.,0.,1.));
#11566=DIRECTION('center_axis',(-1.,0.,0.));
#11567=DIRECTION('ref_axis',(0.,3.46944695195361E-15,1.));
#11568=DIRECTION('',(1.,0.,0.));
#11569=DIRECTION('center_axis',(-1.,0.,0.));
#11570=DIRECTION('ref_axis',(0.,0.,1.));
#11571=DIRECTION('',(-1.,0.,0.));
#11572=DIRECTION('center_axis',(1.,0.,0.));
#11573=DIRECTION('ref_axis',(0.,0.,-1.));
#11574=DIRECTION('',(0.,-1.,3.89551938464967E-15));
#11575=DIRECTION('',(0.,-3.49148133884313E-15,-1.));
#11576=DIRECTION('',(0.,-1.,3.89551938464967E-15));
#11577=DIRECTION('center_axis',(-1.,0.,0.));
#11578=DIRECTION('ref_axis',(0.,0.,1.));
#11579=DIRECTION('',(0.,1.,-3.89551938464967E-15));
#11580=DIRECTION('',(0.,0.,1.));
#11581=DIRECTION('',(0.,1.,-3.89551938464967E-15));
#11582=DIRECTION('center_axis',(0.,-3.89551938464967E-15,-1.));
#11583=DIRECTION('ref_axis',(0.,1.,-3.89551938464967E-15));
#11584=DIRECTION('',(1.,0.,0.));
#11585=DIRECTION('',(0.,1.,0.));
#11586=DIRECTION('',(-0.889029388585716,0.457850135121644,0.));
#11587=DIRECTION('center_axis',(0.,-3.89551938464967E-15,-1.));
#11588=DIRECTION('ref_axis',(0.,1.,-3.89551938464967E-15));
#11589=DIRECTION('',(-0.889029388585716,0.457850135121644,0.));
#11590=DIRECTION('',(0.,1.,0.));
#11591=DIRECTION('',(1.,0.,0.));
#11592=DIRECTION('center_axis',(0.,1.,-3.49148133884313E-15));
#11593=DIRECTION('ref_axis',(0.,3.49148133884313E-15,1.));
#11594=DIRECTION('',(0.,0.,1.));
#11595=DIRECTION('center_axis',(0.457850135121644,0.889029388585716,0.));
#11596=DIRECTION('ref_axis',(-0.889029388585716,0.457850135121644,0.));
#11597=DIRECTION('',(0.,0.,1.));
#11598=DIRECTION('center_axis',(1.,0.,0.));
#11599=DIRECTION('ref_axis',(0.,0.,-1.));
#11600=DIRECTION('center_axis',(-1.,0.,0.));
#11601=DIRECTION('ref_axis',(0.,0.,1.));
#11602=DIRECTION('center_axis',(-1.,0.,0.));
#11603=DIRECTION('ref_axis',(0.,0.,-1.));
#11604=DIRECTION('center_axis',(-1.,0.,0.));
#11605=DIRECTION('ref_axis',(0.,0.,-1.));
#11606=DIRECTION('',(0.,6.98296267768627E-15,-1.));
#11607=DIRECTION('center_axis',(-1.,0.,0.));
#11608=DIRECTION('ref_axis',(0.,0.,1.));
#11609=DIRECTION('center_axis',(1.,0.,0.));
#11610=DIRECTION('ref_axis',(0.,0.,-1.));
#11611=DIRECTION('center_axis',(1.,0.,0.));
#11612=DIRECTION('ref_axis',(0.,0.,-1.));
#11613=DIRECTION('',(0.,6.98296267768627E-15,-1.));
#11614=DIRECTION('center_axis',(1.,0.,0.));
#11615=DIRECTION('ref_axis',(0.,3.46944695195361E-15,-1.));
#11616=DIRECTION('',(-1.,0.,0.));
#11617=DIRECTION('center_axis',(1.,0.,0.));
#11618=DIRECTION('ref_axis',(0.,0.,-1.));
#11619=DIRECTION('',(1.,0.,0.));
#11620=DIRECTION('center_axis',(1.,0.,0.));
#11621=DIRECTION('ref_axis',(0.,0.,-1.));
#11622=DIRECTION('',(0.,1.,3.49148133884313E-15));
#11623=DIRECTION('',(0.,-3.49148133884313E-15,1.));
#11624=DIRECTION('',(0.,1.,3.49148133884313E-15));
#11625=DIRECTION('center_axis',(-1.,0.,0.));
#11626=DIRECTION('ref_axis',(0.,0.,1.));
#11627=DIRECTION('',(0.,-1.,-3.49148133884313E-15));
#11628=DIRECTION('',(0.,3.49148133884313E-15,-1.));
#11629=DIRECTION('',(0.,-1.,-3.49148133884313E-15));
#11630=DIRECTION('center_axis',(0.,-3.49148133884313E-15,1.));
#11631=DIRECTION('ref_axis',(0.,-1.,-3.49148133884313E-15));
#11632=DIRECTION('',(0.889029388585716,-0.457850135121644,-1.59857520276403E-15));
#11633=DIRECTION('',(0.,-1.,-3.49148133884313E-15));
#11634=DIRECTION('',(-1.,0.,0.));
#11635=DIRECTION('center_axis',(0.,-3.49148133884313E-15,1.));
#11636=DIRECTION('ref_axis',(0.,-1.,-3.49148133884313E-15));
#11637=DIRECTION('',(-1.,0.,0.));
#11638=DIRECTION('',(0.,-1.,-3.49148133884313E-15));
#11639=DIRECTION('',(0.889029388585716,-0.457850135121644,-1.59857520276403E-15));
#11640=DIRECTION('center_axis',(0.,1.,3.49148133884313E-15));
#11641=DIRECTION('ref_axis',(0.,-3.49148133884313E-15,1.));
#11642=DIRECTION('',(0.,3.49148133884313E-15,-1.));
#11643=DIRECTION('center_axis',(1.,0.,0.));
#11644=DIRECTION('ref_axis',(0.,0.,-1.));
#11645=DIRECTION('',(0.,3.49148133884313E-15,-1.));
#11646=DIRECTION('center_axis',(0.457850135121644,0.889029388585716,3.10402951993015E-15));
#11647=DIRECTION('ref_axis',(-0.889029388585716,0.457850135121644,4.3777256771857E-32));
#14183=CARTESIAN_POINT('',(0.,0.,0.));
#14184=CARTESIAN_POINT('Origin',(63.9999999999783,34.4999999999999,-2.22044604925031E-13));
#14185=CARTESIAN_POINT('',(57.9999999999783,34.4999999999999,682.31));
#14186=CARTESIAN_POINT('Origin',(63.9999999999783,34.4999999999999,682.31));
#14187=CARTESIAN_POINT('',(57.9999999999783,34.4999999999999,685.31));
#14188=CARTESIAN_POINT('',(57.9999999999783,34.4999999999999,-2.22044604925031E-13));
#14189=CARTESIAN_POINT('Origin',(63.9999999999783,34.4999999999999,685.31));
#14190=CARTESIAN_POINT('Origin',(138.999999999978,34.5,-2.22044604925031E-13));
#14191=CARTESIAN_POINT('',(132.999999999978,34.5,682.31));
#14192=CARTESIAN_POINT('Origin',(138.999999999978,34.5,682.31));
#14193=CARTESIAN_POINT('',(132.999999999978,34.5,685.31));
#14194=CARTESIAN_POINT('',(132.999999999978,34.5,-2.22044604925031E-13));
#14195=CARTESIAN_POINT('Origin',(138.999999999978,34.5,685.31));
#14196=CARTESIAN_POINT('Origin',(63.9999999999783,34.4999999999999,-2.22044604925031E-13));
#14197=CARTESIAN_POINT('',(57.9999999999783,34.4999999999999,-2.22044604925031E-13));
#14198=CARTESIAN_POINT('Origin',(63.9999999999783,34.4999999999999,-2.22044604925031E-13));
#14199=CARTESIAN_POINT('',(57.9999999999783,34.4999999999999,2.99999999999991));
#14200=CARTESIAN_POINT('',(57.9999999999783,34.4999999999999,-2.22044604925031E-13));
#14201=CARTESIAN_POINT('Origin',(63.9999999999783,34.4999999999999,2.99999999999989));
#14202=CARTESIAN_POINT('Origin',(138.999999999978,34.5,-2.22044604925031E-13));
#14203=CARTESIAN_POINT('',(132.999999999978,34.5,-2.22044604925031E-13));
#14204=CARTESIAN_POINT('Origin',(138.999999999978,34.5,-2.22044604925031E-13));
#14205=CARTESIAN_POINT('',(132.999999999978,34.5,2.99999999999991));
#14206=CARTESIAN_POINT('',(132.999999999978,34.5,-2.22044604925031E-13));
#14207=CARTESIAN_POINT('Origin',(138.999999999978,34.5,2.99999999999989));
#14208=CARTESIAN_POINT('Origin',(175.50000000002,4.5,39.4999999999858));
#14209=CARTESIAN_POINT('',(175.50000000002,3.,45.8499999999858));
#14210=CARTESIAN_POINT('Origin',(175.50000000002,3.,39.4999999999858));
#14211=CARTESIAN_POINT('',(175.50000000002,0.,45.8499999999858));
#14212=CARTESIAN_POINT('',(175.50000000002,4.5,45.8499999999858));
#14213=CARTESIAN_POINT('Origin',(175.50000000002,0.,39.4999999999858));
#14214=CARTESIAN_POINT('Origin',(175.500000000001,4.5,645.809999999986));
#14215=CARTESIAN_POINT('',(175.500000000001,3.,652.159999999986));
#14216=CARTESIAN_POINT('Origin',(175.500000000001,3.,645.809999999986));
#14217=CARTESIAN_POINT('',(175.500000000001,0.,652.159999999986));
#14218=CARTESIAN_POINT('',(175.500000000001,4.5,652.159999999986));
#14219=CARTESIAN_POINT('Origin',(175.500000000001,0.,645.809999999986));
#14220=CARTESIAN_POINT('Origin',(32.0000000000012,4.5,39.5000000000189));
#14221=CARTESIAN_POINT('',(32.0000000000012,3.,45.8500000000188));
#14222=CARTESIAN_POINT('Origin',(32.0000000000012,3.,39.5000000000189));
#14223=CARTESIAN_POINT('',(32.0000000000012,0.,45.8500000000188));
#14224=CARTESIAN_POINT('',(32.0000000000012,4.5,45.8500000000188));
#14225=CARTESIAN_POINT('Origin',(32.0000000000012,0.,39.5000000000189));
#14226=CARTESIAN_POINT('Origin',(32.0000000000012,4.5,645.809999999981));
#14227=CARTESIAN_POINT('',(32.0000000000012,3.,652.159999999981));
#14228=CARTESIAN_POINT('Origin',(32.0000000000012,3.,645.809999999981));
#14229=CARTESIAN_POINT('',(32.0000000000012,0.,652.159999999981));
#14230=CARTESIAN_POINT('',(32.0000000000012,4.5,652.159999999981));
#14231=CARTESIAN_POINT('Origin',(32.0000000000012,0.,645.809999999981));
#14232=CARTESIAN_POINT('Origin',(134.030507120984,66.,0.));
#14233=CARTESIAN_POINT('',(134.030507120984,66.,0.));
#14234=CARTESIAN_POINT('',(134.030507120984,66.,0.127016653792582));
#14235=CARTESIAN_POINT('',(134.030507120984,66.,0.));
#14236=CARTESIAN_POINT('',(134.030507120984,69.,4.));
#14237=CARTESIAN_POINT('Origin',(134.030507120984,65.,4.));
#14238=CARTESIAN_POINT('',(134.030507120984,69.,1.83697019872103E-16));
#14239=CARTESIAN_POINT('',(134.030507120984,69.,685.31));
#14240=CARTESIAN_POINT('',(134.030507120984,69.,0.));
#14241=CARTESIAN_POINT('Origin',(4.,66.,4.));
#14242=CARTESIAN_POINT('',(4.,69.,4.));
#14243=CARTESIAN_POINT('',(4.,69.,1.83697019872103E-16));
#14244=CARTESIAN_POINT('',(4.00000000000059,69.,685.31));
#14245=CARTESIAN_POINT('',(4.,66.,0.127016653792582));
#14246=CARTESIAN_POINT('Origin',(4.,65.,4.));
#14247=CARTESIAN_POINT('',(4.,66.,0.));
#14248=CARTESIAN_POINT('',(4.,66.,4.));
#14249=CARTESIAN_POINT('',(4.,66.,0.));
#14250=CARTESIAN_POINT('Origin',(0.,69.,685.31));
#14251=CARTESIAN_POINT('',(134.030507120984,68.9999999999999,681.31));
#14252=CARTESIAN_POINT('',(134.030507120984,69.,685.31));
#14253=CARTESIAN_POINT('',(134.030507120984,69.,4.));
#14254=CARTESIAN_POINT('',(4.,68.9999999999999,681.31));
#14255=CARTESIAN_POINT('',(4.,69.,685.31));
#14256=CARTESIAN_POINT('',(4.,68.9999999999999,681.31));
#14257=CARTESIAN_POINT('Origin',(0.,66.,685.31));
#14258=CARTESIAN_POINT('',(134.030507120984,66.,4.));
#14259=CARTESIAN_POINT('',(4.,66.,4.));
#14260=CARTESIAN_POINT('',(134.030507120984,66.,4.));
#14261=CARTESIAN_POINT('',(134.030507120984,66.,681.31));
#14262=CARTESIAN_POINT('',(134.030507120984,66.,685.31));
#14263=CARTESIAN_POINT('',(4.,65.9999999999999,681.31));
#14264=CARTESIAN_POINT('',(4.,65.9999999999999,681.31));
#14265=CARTESIAN_POINT('',(4.,66.,685.31));
#14266=CARTESIAN_POINT('Origin',(4.,66.,685.31));
#14267=CARTESIAN_POINT('',(4.,66.,685.31));
#14268=CARTESIAN_POINT('',(4.,66.,685.182983346207));
#14269=CARTESIAN_POINT('',(4.,66.,685.31));
#14270=CARTESIAN_POINT('Origin',(4.,64.9999999999999,681.31));
#14271=CARTESIAN_POINT('',(4.,69.,685.31));
#14272=CARTESIAN_POINT('',(4.,69.,685.31));
#14273=CARTESIAN_POINT('',(4.,69.,685.31));
#14274=CARTESIAN_POINT('Origin',(134.030507120984,65.9999999999999,681.31));
#14275=CARTESIAN_POINT('',(134.030507120984,69.,685.31));
#14276=CARTESIAN_POINT('',(134.030507120984,69.,685.31));
#14277=CARTESIAN_POINT('',(134.030507120984,66.,685.182983346207));
#14278=CARTESIAN_POINT('Origin',(134.030507120984,64.9999999999999,681.31));
#14279=CARTESIAN_POINT('',(134.030507120984,66.,685.31));
#14280=CARTESIAN_POINT('',(134.030507120984,66.,685.31));
#14281=CARTESIAN_POINT('',(134.030507120984,66.,685.31));
#14282=CARTESIAN_POINT('Origin',(0.,4.,685.31));
#14283=CARTESIAN_POINT('',(0.,4.,685.31));
#14284=CARTESIAN_POINT('',(3.,4.,685.31));
#14285=CARTESIAN_POINT('',(0.,4.,685.31));
#14286=CARTESIAN_POINT('',(4.,0.,685.31));
#14287=CARTESIAN_POINT('Origin',(4.,4.,685.31));
#14288=CARTESIAN_POINT('',(4.,3.,685.31));
#14289=CARTESIAN_POINT('',(4.,3.,685.31));
#14290=CARTESIAN_POINT('Origin',(4.,4.,685.31));
#14291=CARTESIAN_POINT('Origin',(4.,3.,685.31));
#14292=CARTESIAN_POINT('',(0.,65.,685.31));
#14293=CARTESIAN_POINT('',(0.,0.,685.31));
#14294=CARTESIAN_POINT('',(3.,65.,685.31));
#14295=CARTESIAN_POINT('',(3.,0.,685.31));
#14296=CARTESIAN_POINT('',(3.,65.,685.31));
#14297=CARTESIAN_POINT('Origin',(4.,0.,0.));
#14298=CARTESIAN_POINT('',(4.,0.,0.));
#14299=CARTESIAN_POINT('',(4.,3.,0.));
#14300=CARTESIAN_POINT('',(4.,0.,0.));
#14301=CARTESIAN_POINT('',(0.,4.,0.));
#14302=CARTESIAN_POINT('Origin',(4.,4.,0.));
#14303=CARTESIAN_POINT('',(3.,4.,0.));
#14304=CARTESIAN_POINT('',(3.,4.,0.));
#14305=CARTESIAN_POINT('Origin',(4.,4.,0.));
#14306=CARTESIAN_POINT('Origin',(3.,4.,0.));
#14307=CARTESIAN_POINT('',(60.,0.,0.));
#14308=CARTESIAN_POINT('',(0.,0.,0.));
#14309=CARTESIAN_POINT('',(60.,3.,0.));
#14310=CARTESIAN_POINT('',(0.,3.,0.));
#14311=CARTESIAN_POINT('',(60.,3.,0.));
#14312=CARTESIAN_POINT('Origin',(4.,69.,685.31));
#14313=CARTESIAN_POINT('Origin',(4.,65.,685.31));
#14314=CARTESIAN_POINT('Origin',(4.,65.,685.31));
#14315=CARTESIAN_POINT('Origin',(0.,65.,0.));
#14316=CARTESIAN_POINT('',(0.,65.,0.));
#14317=CARTESIAN_POINT('',(3.,65.,0.));
#14318=CARTESIAN_POINT('',(0.,65.,0.));
#14319=CARTESIAN_POINT('Origin',(4.,65.,0.));
#14320=CARTESIAN_POINT('Origin',(4.,65.,0.));
#14321=CARTESIAN_POINT('Origin',(4.,66.,0.));
#14322=CARTESIAN_POINT('',(0.,0.,0.));
#14323=CARTESIAN_POINT('',(3.,0.,0.));
#14324=CARTESIAN_POINT('Origin',(135.86190766147,68.5561175543429,685.31));
#14325=CARTESIAN_POINT('',(135.86190766147,68.5561175543429,685.31));
#14326=CARTESIAN_POINT('',(134.488357256105,65.8890293885857,685.31));
#14327=CARTESIAN_POINT('',(135.86190766147,68.5561175543429,685.31));
#14328=CARTESIAN_POINT('Origin',(134.030507120984,65.,685.31));
#14329=CARTESIAN_POINT('Origin',(134.030507120984,65.,685.31));
#14330=CARTESIAN_POINT('Origin',(134.030507120984,66.,685.31));
#14331=CARTESIAN_POINT('',(192.831400540487,39.2168287216494,685.31));
#14332=CARTESIAN_POINT('',(135.,69.,685.31));
#14333=CARTESIAN_POINT('',(191.457850135122,36.5497405558923,685.31));
#14334=CARTESIAN_POINT('',(133.626449594635,66.3329118342429,685.31));
#14335=CARTESIAN_POINT('',(191.457850135122,36.5497405558923,685.31));
#14336=CARTESIAN_POINT('Origin',(134.030507120984,69.,0.));
#14337=CARTESIAN_POINT('',(135.86190766147,68.5561175543429,0.));
#14338=CARTESIAN_POINT('Origin',(134.030507120984,65.,0.));
#14339=CARTESIAN_POINT('',(134.488357256105,65.8890293885857,0.));
#14340=CARTESIAN_POINT('',(134.488357256105,65.8890293885857,0.));
#14341=CARTESIAN_POINT('Origin',(134.030507120984,65.,0.));
#14342=CARTESIAN_POINT('Origin',(195.,35.6607111673066,685.31));
#14343=CARTESIAN_POINT('',(195.,35.6607111673066,685.31));
#14344=CARTESIAN_POINT('',(192.,35.6607111673066,685.31));
#14345=CARTESIAN_POINT('',(195.,35.6607111673066,685.31));
#14346=CARTESIAN_POINT('Origin',(191.,35.6607111673066,685.31));
#14347=CARTESIAN_POINT('Origin',(191.,35.6607111673066,685.31));
#14348=CARTESIAN_POINT('Origin',(191.457850135122,36.5497405558923,685.31));
#14349=CARTESIAN_POINT('',(195.,4.00000000000003,685.31));
#14350=CARTESIAN_POINT('',(195.,38.1,685.31));
#14351=CARTESIAN_POINT('',(192.,4.00000000000001,685.31));
#14352=CARTESIAN_POINT('',(192.,38.1,685.31));
#14353=CARTESIAN_POINT('',(192.,4.00000000000001,685.31));
#14354=CARTESIAN_POINT('Origin',(192.831400540487,39.2168287216494,0.));
#14355=CARTESIAN_POINT('',(192.831400540487,39.2168287216494,0.));
#14356=CARTESIAN_POINT('',(191.457850135122,36.5497405558923,0.));
#14357=CARTESIAN_POINT('',(192.831400540487,39.2168287216494,0.));
#14358=CARTESIAN_POINT('',(195.,35.6607111673066,0.));
#14359=CARTESIAN_POINT('Origin',(191.,35.6607111673066,0.));
#14360=CARTESIAN_POINT('',(192.,35.6607111673066,0.));
#14361=CARTESIAN_POINT('',(192.,35.6607111673066,0.));
#14362=CARTESIAN_POINT('Origin',(191.,35.6607111673066,0.));
#14363=CARTESIAN_POINT('Origin',(192.,35.6607111673066,0.));
#14364=CARTESIAN_POINT('',(135.,69.,0.));
#14365=CARTESIAN_POINT('',(133.626449594635,66.3329118342429,0.));
#14366=CARTESIAN_POINT('Origin',(191.,-4.89858719658945E-16,685.31));
#14367=CARTESIAN_POINT('',(191.,-4.89858719658945E-16,685.31));
#14368=CARTESIAN_POINT('',(191.,3.,685.31));
#14369=CARTESIAN_POINT('',(191.,-4.89858719658945E-16,685.31));
#14370=CARTESIAN_POINT('Origin',(191.,4.00000000000001,685.31));
#14371=CARTESIAN_POINT('Origin',(191.,4.00000000000001,685.31));
#14372=CARTESIAN_POINT('Origin',(192.,4.00000000000001,685.31));
#14373=CARTESIAN_POINT('',(160.,-4.28626379701574E-15,685.31));
#14374=CARTESIAN_POINT('',(195.,-3.08148791101958E-30,685.31));
#14375=CARTESIAN_POINT('',(160.,3.,685.31));
#14376=CARTESIAN_POINT('',(195.,3.,685.31));
#14377=CARTESIAN_POINT('',(160.,-4.28626379701574E-15,685.31));
#14378=CARTESIAN_POINT('Origin',(195.,4.00000000000003,0.));
#14379=CARTESIAN_POINT('',(195.,4.00000000000003,0.));
#14380=CARTESIAN_POINT('',(192.,4.00000000000001,0.));
#14381=CARTESIAN_POINT('',(195.,4.00000000000003,0.));
#14382=CARTESIAN_POINT('',(191.,-4.89858719658945E-16,0.));
#14383=CARTESIAN_POINT('Origin',(191.,4.00000000000001,0.));
#14384=CARTESIAN_POINT('',(191.,3.,0.));
#14385=CARTESIAN_POINT('',(191.,3.,0.));
#14386=CARTESIAN_POINT('Origin',(191.,4.00000000000001,0.));
#14387=CARTESIAN_POINT('Origin',(191.,3.,0.));
#14388=CARTESIAN_POINT('',(195.,38.1,0.));
#14389=CARTESIAN_POINT('',(192.,38.1,0.));
#14390=CARTESIAN_POINT('Origin',(195.,3.,685.31));
#14391=CARTESIAN_POINT('',(160.,3.,0.));
#14392=CARTESIAN_POINT('',(195.,3.,0.));
#14393=CARTESIAN_POINT('',(160.,3.,685.31));
#14394=CARTESIAN_POINT('',(191.,3.,685.31));
#14395=CARTESIAN_POINT('Origin',(160.,-4.28626379701574E-15,685.31));
#14396=CARTESIAN_POINT('',(160.,-4.28626379701574E-15,0.));
#14397=CARTESIAN_POINT('',(160.,-4.28626379701574E-15,0.));
#14398=CARTESIAN_POINT('',(160.,-4.28626379701574E-15,685.31));
#14399=CARTESIAN_POINT('Origin',(195.,-3.08148791101958E-30,685.31));
#14400=CARTESIAN_POINT('',(195.,-3.08148791101958E-30,0.));
#14401=CARTESIAN_POINT('',(191.,-4.89858719658945E-16,685.31));
#14402=CARTESIAN_POINT('Origin',(191.,4.00000000000001,685.31));
#14403=CARTESIAN_POINT('',(195.,4.00000000000003,685.31));
#14404=CARTESIAN_POINT('Origin',(195.,38.1,685.31));
#14405=CARTESIAN_POINT('',(195.,35.6607111673066,685.31));
#14406=CARTESIAN_POINT('Origin',(191.,35.6607111673066,685.31));
#14407=CARTESIAN_POINT('',(192.831400540487,39.2168287216494,685.31));
#14408=CARTESIAN_POINT('Origin',(135.,69.,685.31));
#14409=CARTESIAN_POINT('',(135.86190766147,68.5561175543429,685.31));
#14410=CARTESIAN_POINT('Origin',(134.030507120984,65.,685.31));
#14411=CARTESIAN_POINT('Origin',(4.,65.,685.31));
#14412=CARTESIAN_POINT('',(0.,65.,685.31));
#14413=CARTESIAN_POINT('Origin',(0.,0.,685.31));
#14414=CARTESIAN_POINT('',(0.,4.,685.31));
#14415=CARTESIAN_POINT('Origin',(4.,4.,685.31));
#14416=CARTESIAN_POINT('',(4.,0.,685.31));
#14417=CARTESIAN_POINT('Origin',(0.,0.,685.31));
#14418=CARTESIAN_POINT('',(60.,0.,685.31));
#14419=CARTESIAN_POINT('',(60.,0.,685.31));
#14420=CARTESIAN_POINT('',(0.,0.,685.31));
#14421=CARTESIAN_POINT('Origin',(60.,3.,685.31));
#14422=CARTESIAN_POINT('',(60.,3.,685.31));
#14423=CARTESIAN_POINT('',(60.,3.,685.31));
#14424=CARTESIAN_POINT('',(60.,3.,685.31));
#14425=CARTESIAN_POINT('Origin',(0.,3.,685.31));
#14426=CARTESIAN_POINT('',(4.,3.,685.31));
#14427=CARTESIAN_POINT('',(0.,3.,685.31));
#14428=CARTESIAN_POINT('Origin',(4.,4.,685.31));
#14429=CARTESIAN_POINT('',(3.,4.,685.31));
#14430=CARTESIAN_POINT('Origin',(3.,0.,685.31));
#14431=CARTESIAN_POINT('',(3.,65.,685.31));
#14432=CARTESIAN_POINT('Origin',(4.,65.,685.31));
#14433=CARTESIAN_POINT('',(4.,66.,4.));
#14434=CARTESIAN_POINT('',(4.,66.,685.31));
#14435=CARTESIAN_POINT('Origin',(134.030507120984,65.,685.31));
#14436=CARTESIAN_POINT('',(134.488357256105,65.8890293885857,685.31));
#14437=CARTESIAN_POINT('',(134.030507120984,66.,685.31));
#14438=CARTESIAN_POINT('',(134.030507120984,66.,0.));
#14439=CARTESIAN_POINT('Origin',(133.626449594635,66.3329118342429,685.31));
#14440=CARTESIAN_POINT('',(191.457850135122,36.5497405558923,685.31));
#14441=CARTESIAN_POINT('Origin',(191.,35.6607111673066,685.31));
#14442=CARTESIAN_POINT('',(192.,35.6607111673066,685.31));
#14443=CARTESIAN_POINT('Origin',(192.,38.1,685.31));
#14444=CARTESIAN_POINT('',(192.,4.00000000000001,685.31));
#14445=CARTESIAN_POINT('Origin',(191.,4.00000000000001,685.31));
#14446=CARTESIAN_POINT('Origin',(191.,4.00000000000001,685.31));
#14447=CARTESIAN_POINT('Origin',(191.,4.00000000000001,0.));
#14448=CARTESIAN_POINT('Origin',(134.030507120984,64.9999999999999,681.31));
#14449=CARTESIAN_POINT('',(134.030507120984,64.9999999999999,685.31));
#14450=CARTESIAN_POINT('Origin',(134.030507120984,64.9999999999999,681.31));
#14451=CARTESIAN_POINT('',(134.030507120984,64.9999999999999,682.31));
#14452=CARTESIAN_POINT('',(134.030507120984,64.9999999999999,685.31));
#14453=CARTESIAN_POINT('Origin',(134.030507120984,64.9999999999999,681.31));
#14454=CARTESIAN_POINT('Origin',(4.,64.9999999999999,681.31));
#14455=CARTESIAN_POINT('',(4.,64.9999999999999,685.31));
#14456=CARTESIAN_POINT('Origin',(4.,64.9999999999999,681.31));
#14457=CARTESIAN_POINT('',(4.,64.9999999999999,682.31));
#14458=CARTESIAN_POINT('Origin',(4.,64.9999999999999,681.31));
#14459=CARTESIAN_POINT('',(4.,64.9999999999999,682.31));
#14460=CARTESIAN_POINT('Origin',(4.,64.9999999999999,681.31));
#14461=CARTESIAN_POINT('',(134.030507120984,64.9999999999999,685.31));
#14462=CARTESIAN_POINT('Origin',(4.,64.9999999999999,681.31));
#14463=CARTESIAN_POINT('',(134.030507120984,64.9999999999999,682.31));
#14464=CARTESIAN_POINT('Origin',(4.,9.00000000000001,685.31));
#14465=CARTESIAN_POINT('',(4.,8.99999999999999,682.31));
#14466=CARTESIAN_POINT('',(4.,8.99999999999999,682.31));
#14467=CARTESIAN_POINT('',(4.,9.00000000000001,685.31));
#14468=CARTESIAN_POINT('',(4.,9.00000000000001,685.31));
#14469=CARTESIAN_POINT('',(4.,2.6801128335108E-12,685.31));
#14470=CARTESIAN_POINT('Origin',(134.030507120984,66.,685.31));
#14471=CARTESIAN_POINT('',(134.030507120984,61.3121699873772,685.31));
#14472=CARTESIAN_POINT('',(134.030507120984,2.6801128335108E-12,685.31));
#14473=CARTESIAN_POINT('',(134.030507120984,61.3121699873772,682.31));
#14474=CARTESIAN_POINT('',(134.030507120984,61.3121699873772,682.31));
#14475=CARTESIAN_POINT('',(134.030507120984,66.,682.31));
#14476=CARTESIAN_POINT('Origin',(0.,2.6801128335108E-12,685.31));
#14477=CARTESIAN_POINT('',(187.353206910234,9.00000000000001,685.31));
#14478=CARTESIAN_POINT('',(0.,9.00000000000001,685.31));
#14479=CARTESIAN_POINT('',(187.353206910234,33.8509795959131,685.31));
#14480=CARTESIAN_POINT('',(187.353206910234,9.00000000000001,685.31));
#14481=CARTESIAN_POINT('',(187.353206910234,33.8509795959131,685.31));
#14482=CARTESIAN_POINT('Origin',(0.,2.66963838949427E-12,682.31));
#14483=CARTESIAN_POINT('',(187.353206910234,33.8509795959131,682.31));
#14484=CARTESIAN_POINT('',(187.353206910234,33.8509795959131,682.31));
#14485=CARTESIAN_POINT('',(187.353206910234,9.00000000000001,682.31));
#14486=CARTESIAN_POINT('',(187.353206910234,9.00000000000001,682.31));
#14487=CARTESIAN_POINT('',(134.030507120984,8.99999999999999,682.31));
#14488=CARTESIAN_POINT('Origin',(134.030507120984,9.00000000000001,685.31));
#14489=CARTESIAN_POINT('',(187.353206910234,9.00000000000001,682.31));
#14490=CARTESIAN_POINT('Origin',(187.353206910234,33.8509795959131,682.31));
#14491=CARTESIAN_POINT('',(187.353206910234,33.8509795959131,682.31));
#14492=CARTESIAN_POINT('Origin',(187.353206910234,9.00000000000001,682.31));
#14493=CARTESIAN_POINT('Origin',(4.,65.,4.));
#14494=CARTESIAN_POINT('',(4.,65.,3.));
#14495=CARTESIAN_POINT('Origin',(4.,65.,4.));
#14496=CARTESIAN_POINT('',(4.,65.,-1.73472347597681E-15));
#14497=CARTESIAN_POINT('Origin',(4.,65.,4.));
#14498=CARTESIAN_POINT('',(4.,65.,-6.98296267768613E-15));
#14499=CARTESIAN_POINT('Origin',(134.030507120984,65.,4.));
#14500=CARTESIAN_POINT('',(134.030507120984,65.,-3.328228599496E-15));
#14501=CARTESIAN_POINT('Origin',(134.030507120984,65.,4.));
#14502=CARTESIAN_POINT('',(134.030507120984,65.,3.));
#14503=CARTESIAN_POINT('Origin',(134.030507120984,65.,4.));
#14504=CARTESIAN_POINT('',(134.030507120984,65.,3.));
#14505=CARTESIAN_POINT('Origin',(134.030507120984,65.,4.));
#14506=CARTESIAN_POINT('',(4.,65.,-3.46944695195361E-15));
#14507=CARTESIAN_POINT('Origin',(134.030507120984,65.,4.));
#14508=CARTESIAN_POINT('',(4.,65.,3.));
#14509=CARTESIAN_POINT('Origin',(4.,66.,0.));
#14510=CARTESIAN_POINT('',(4.,9.00000000000001,-1.98861209386333E-13));
#14511=CARTESIAN_POINT('',(4.,1.04744440165302E-14,-2.30284541435921E-13));
#14512=CARTESIAN_POINT('',(4.,8.99999999999999,2.9999999999998));
#14513=CARTESIAN_POINT('',(4.,9.00000000000001,-1.99014436314059E-13));
#14514=CARTESIAN_POINT('',(4.,66.,3.));
#14515=CARTESIAN_POINT('Origin',(134.030507120984,9.00000000000001,-1.99059518868339E-13));
#14516=CARTESIAN_POINT('',(134.030507120984,61.3121699873795,3.00000000000021));
#14517=CARTESIAN_POINT('',(134.030507120984,8.99999999999999,2.9999999999998));
#14518=CARTESIAN_POINT('',(134.030507120984,61.3121699873796,2.14070297354914E-13));
#14519=CARTESIAN_POINT('',(134.030507120984,61.3121699873795,3.00000000000021));
#14520=CARTESIAN_POINT('',(134.030507120984,1.04744440165302E-14,-2.30284541435921E-13));
#14521=CARTESIAN_POINT('Origin',(0.,1.04744440165302E-14,-2.30284541435921E-13));
#14522=CARTESIAN_POINT('',(187.353206910234,33.8509795959155,1.18190063560699E-13));
#14523=CARTESIAN_POINT('',(134.030507120984,61.3121699873796,2.14070297354914E-13));
#14524=CARTESIAN_POINT('',(187.353206910234,9.0000000000024,3.14233320495966E-14));
#14525=CARTESIAN_POINT('',(187.353206910234,33.8509795959155,1.18190063560699E-13));
#14526=CARTESIAN_POINT('',(0.,9.00000000000001,-1.98861209386333E-13));
#14527=CARTESIAN_POINT('Origin',(0.,8.04569168006329E-28,2.99999999999977));
#14528=CARTESIAN_POINT('',(187.353206910234,9.00000000000239,3.00000000000003));
#14529=CARTESIAN_POINT('',(4.,8.99999999999999,2.9999999999998));
#14530=CARTESIAN_POINT('',(187.353206910234,33.8509795959155,3.00000000000012));
#14531=CARTESIAN_POINT('',(187.353206910234,33.8509795959155,3.00000000000012));
#14532=CARTESIAN_POINT('',(134.030507120984,61.3121699873795,3.00000000000021));
#14533=CARTESIAN_POINT('Origin',(4.,9.00000000000001,-1.99059518868339E-13));
#14534=CARTESIAN_POINT('',(187.353206910234,9.00000000000239,3.00000000000003));
#14535=CARTESIAN_POINT('Origin',(187.353206910234,33.8509795959155,3.00000000000012));
#14536=CARTESIAN_POINT('',(187.353206910234,33.8509795959155,3.00000000000012));
#14537=CARTESIAN_POINT('Origin',(134.030507120984,61.3121699873795,3.00000000000021));
#17969=UNCERTAINTY_MEASURE_WITH_UNIT(LENGTH_MEASURE(0.01),#18007,
'DISTANCE_ACCURACY_VALUE',
'Maximum model space distance between geometric entities at asserted c
onnectivities');
#17986=UNCERTAINTY_MEASURE_WITH_UNIT(LENGTH_MEASURE(0.01),#18007,
'DISTANCE_ACCURACY_VALUE',
'Maximum model space distance between geometric entities at asserted c
onnectivities');
#17989=(
GEOMETRIC_REPRESENTATION_CONTEXT(3)
GLOBAL_UNCERTAINTY_ASSIGNED_CONTEXT((#17969))
GLOBAL_UNIT_ASSIGNED_CONTEXT((#18007,#18009,#18010))
REPRESENTATION_CONTEXT('','3D')
);
#18006=(
GEOMETRIC_REPRESENTATION_CONTEXT(3)
GLOBAL_UNCERTAINTY_ASSIGNED_CONTEXT((#17986))
GLOBAL_UNIT_ASSIGNED_CONTEXT((#18007,#18009,#18010))
REPRESENTATION_CONTEXT('','3D')
);
#18007=(
LENGTH_UNIT()
NAMED_UNIT(*)
SI_UNIT(.MILLI.,.METRE.)
);
#18009=(
NAMED_UNIT(*)
PLANE_ANGLE_UNIT()
SI_UNIT($,.RADIAN.)
);
#18010=(
NAMED_UNIT(*)
SI_UNIT($,.STERADIAN.)
SOLID_ANGLE_UNIT()
);
#18013=SHAPE_DEFINITION_REPRESENTATION(#18032,#18072);
#18032=PRODUCT_DEFINITION_SHAPE('',$,#18092);
#18072=SHAPE_REPRESENTATION('',(#9886),#17989);
#18089=PRODUCT_DEFINITION_CONTEXT('part definition',#18148,'design');
#18092=PRODUCT_DEFINITION('Top Rail','Top Rail',#18111,#18089);
#18111=PRODUCT_DEFINITION_FORMATION('',$,#18152);
#18148=APPLICATION_CONTEXT(
'Core Data for Automotive Mechanical Design Process');
#18149=PRODUCT_CONTEXT('part definition',#18148,'mechanical');
#18152=PRODUCT('Top Rail','Top Rail',$,(#18149));
#18170=PRESENTATION_STYLE_ASSIGNMENT((#18174));
#18174=SURFACE_STYLE_USAGE(.BOTH.,#18178);
#18178=SURFACE_SIDE_STYLE('',(#18182));
#18182=SURFACE_STYLE_FILL_AREA(#18186);
#18186=FILL_AREA_STYLE('Opaque(227,224,212)',(#18190));
#18190=FILL_AREA_STYLE_COLOUR('Opaque(227,224,212)',#18194);
#18194=COLOUR_RGB('Opaque(227,224,212)',0.890196078431372,0.87843137254902,
0.831372549019608);
ENDSEC;
END-ISO-10303-21;
